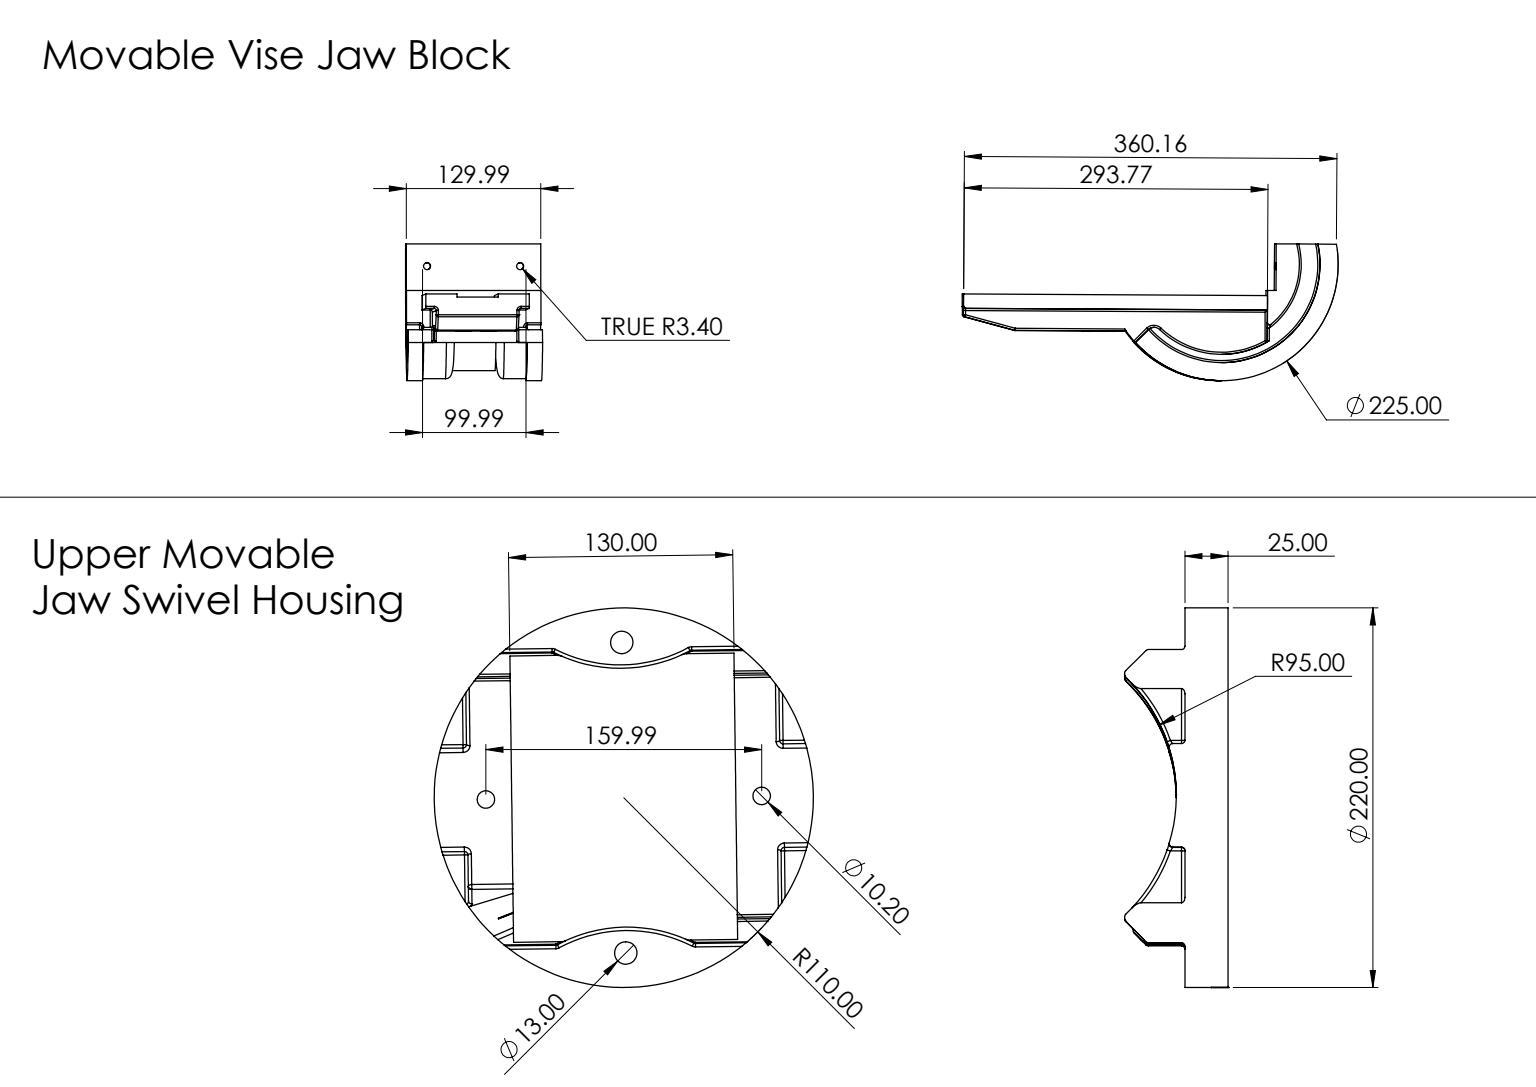
ISO-10303-21;
HEADER;
FILE_DESCRIPTION (('STEP AP214'),
    '1' );
FILE_NAME ('Movable Vise Jaw Block.step',
    '2026-10-09T10:51:02',
    ( '' ),
    ( '' ),
    'SwSTEP 2.0',
    'SolidWorks 2026',
    '' );
FILE_SCHEMA (( 'AUTOMOTIVE_DESIGN' ));
ENDSEC;

DATA;
#3=FACE_BOUND ( 'NONE', #13638, .T. ) ;
#7=LINE ( 'NONE', #21024, #14851 ) ;
#9=DIRECTION ( 'NONE',  ( 0.01292394549866739996, 0.005513023399721564584, 0.9999012842304692006 ) ) ;
#20=DIRECTION ( 'NONE',  ( 0.9999164797902017066, 6.965998958219365988E-18, -0.01292414190464157356 ) ) ;
#23=ORIENTED_EDGE ( 'NONE', *, *, #4860, .T. ) ;
#32=EDGE_CURVE ( 'NONE', #7434, #9119, #18827, .T. ) ;
#56=CARTESIAN_POINT ( 'NONE',  ( -66.42677970909001317, 189.3893605493459233, -109.9672025422466959 ) ) ;
#62=EDGE_CURVE ( 'NONE', #12374, #18464, #11714, .T. ) ;
#74=ORIENTED_EDGE ( 'NONE', *, *, #20006, .F. ) ;
#82=AXIS2_PLACEMENT_3D ( 'NONE', #13509, #3038, #10060 ) ;
#96=CARTESIAN_POINT ( 'NONE',  ( -45.67464185259402853, 168.2105890667581605, -51.90496219196452188 ) ) ;
#109=DIRECTION ( 'NONE',  ( -0.01292394549866736179, -0.005513023399728320464, -0.9999012842304692006 ) ) ;
#113=CONICAL_SURFACE ( 'NONE', #10017, 3.399999999999985700, 1.029744258676653201 ) ;
#115=ORIENTED_EDGE ( 'NONE', *, *, #3028, .T. ) ;
#117=CARTESIAN_POINT ( 'NONE',  ( -39.93340742419142941, 174.9483409995870886, 5.410635606648346752 ) ) ;
#119=CARTESIAN_POINT ( 'NONE',  ( -49.95600144165727841, 95.32463374251413768, -43.99660977802226114 ) ) ;
#124=CIRCLE ( 'NONE', #10026, 112.5000000000000142 ) ;
#136=AXIS2_PLACEMENT_3D ( 'NONE', #9103, #21501, #2221 ) ;
#140=DIRECTION ( 'NONE',  ( 0.9999164797902015955, 6.965998958219364448E-18, -0.01292414190464157182 ) ) ;
#141=CARTESIAN_POINT ( 'NONE',  ( 43.08423624159371457, 94.48610424851698042, 82.84014869562157912 ) ) ;
#148=CARTESIAN_POINT ( 'NONE',  ( -65.67129704762463405, 144.7109461922390778, -51.51693412452669918 ) ) ;
#149=AXIS2_PLACEMENT_3D ( 'NONE', #2906, #22065, #6366 ) ;
#163=VERTEX_POINT ( 'NONE', #8594 ) ;
#169=EDGE_CURVE ( 'NONE', #21645, #1999, #4525, .T. ) ;
#175=VECTOR ( 'NONE', #4968, 999.9999999999998863 ) ;
#178=CARTESIAN_POINT ( 'NONE',  ( -38.71484115365228007, 95.23700578170286235, 83.13812943312275650 ) ) ;
#185=CARTESIAN_POINT ( 'NONE',  ( -10.80196055862741211, 113.7230284608895943, 131.4548877534794542 ) ) ;
#187=ORIENTED_EDGE ( 'NONE', *, *, #11712, .T. ) ;
#193=CIRCLE ( 'NONE', #21802, 95.00000000000001421 ) ;
#208=ADVANCED_FACE ( 'NONE', ( #17222 ), #15410, .F. ) ;
#212=AXIS2_PLACEMENT_3D ( 'NONE', #480, #21365, #21476 ) ;
#229=ORIENTED_EDGE ( 'NONE', *, *, #7447, .T. ) ;
#238=DIRECTION ( 'NONE',  ( 0.01246513159389400598, 0.2641402835564878870, 0.9644037178988087433 ) ) ;
#241=ORIENTED_EDGE ( 'NONE', *, *, #10232, .T. ) ;
#242=CARTESIAN_POINT ( 'NONE',  ( -29.42617654240078551, 169.3906321239456361, -110.1596432836334856 ) ) ;
#245=ORIENTED_EDGE ( 'NONE', *, *, #7257, .T. ) ;
#257=ORIENTED_EDGE ( 'NONE', *, *, #16631, .F. ) ;
#262=DIRECTION ( 'NONE',  ( -0.01292394549866739996, -0.005513023399721131770, -0.9999012842304692006 ) ) ;
#263=CARTESIAN_POINT ( 'NONE',  ( -39.11958398656035030, 107.9174803907495885, 72.42004164600064087 ) ) ;
#264=DIRECTION ( 'NONE',  ( -7.125109674159588039E-05, 0.9999848031710253382, -0.005512562950848870491 ) ) ;
#269=EDGE_LOOP ( 'NONE', ( #10049, #17678 ) ) ;
#276=FACE_OUTER_BOUND ( 'NONE', #812, .T. ) ;
#280=CARTESIAN_POINT ( 'NONE',  ( -38.57134427488318806, 95.07266577213218284, 83.30245068639356987 ) ) ;
#286=ORIENTED_EDGE ( 'NONE', *, *, #7951, .T. ) ;
#292=EDGE_CURVE ( 'NONE', #16435, #21883, #7077, .T. ) ;
#296=B_SPLINE_CURVE_WITH_KNOTS ( 'NONE', 3,
 ( #20681, #1405, #18731, #13805, #4936, #18621, #1059, #11969, #4819, #17038, #18953, #20788, #17137, #20446, #8179, #13473 ),
 .UNSPECIFIED., .F., .F.,
 ( 4, 2, 2, 2, 2, 2, 2, 4 ),
 ( 0.000000000000000000, 0.0008474927940828290429, 0.001271239191124224699, 0.001694985588165620572, 0.002118731985207016229, 0.002542478382248412102, 0.002966224779289807541, 0.003389971176331203415 ),
 .UNSPECIFIED. ) ;
#302=DIRECTION ( 'NONE',  ( 0.01292394549866740169, 0.005513023399720822990, 0.9999012842304693116 ) ) ;
#309=VERTEX_POINT ( 'NONE', #21424 ) ;
#311=DIRECTION ( 'NONE',  ( 0.01292394549866739996, 0.005513023399721131770, 0.9999012842304692006 ) ) ;
#312=EDGE_LOOP ( 'NONE', ( #22638, #21700, #16864 ) ) ;
#329=CIRCLE ( 'NONE', #7287, 112.5000000000000284 ) ;
#332=VECTOR ( 'NONE', #8959, 1000.000000000000114 ) ;
#335=CARTESIAN_POINT ( 'NONE',  ( -66.44851505496320954, 169.3797848675314128, -111.6488252521261160 ) ) ;
#336=LINE ( 'NONE', #12856, #8327 ) ;
#338=CARTESIAN_POINT ( 'NONE',  ( -50.59154831888564274, 96.21415597129798414, -45.44386052779758245 ) ) ;
#340=CARTESIAN_POINT ( 'NONE',  ( -48.94038278341281512, 95.51270090492249665, 82.30370228625183415 ) ) ;
#344=ORIENTED_EDGE ( 'NONE', *, *, #10316, .T. ) ;
#346=CARTESIAN_POINT ( 'NONE',  ( 40.57355171551004958, 108.0982075334647163, 198.8652726751216449 ) ) ;
#374=CYLINDRICAL_SURFACE ( 'NONE', #1941, 2.000000000000001332 ) ;
#375=DIRECTION ( 'NONE',  ( 0.01292394549866743812, 0.005513023399720639109, 0.9999012842304693116 ) ) ;
#376=AXIS2_PLACEMENT_3D ( 'NONE', #2393, #7090, #10992 ) ;
#384=VECTOR ( 'NONE', #9453, 1000.000000000000000 ) ;
#395=CARTESIAN_POINT ( 'NONE',  ( -38.29718547875438617, 94.85299739018206822, 83.52102959496109236 ) ) ;
#411=ORIENTED_EDGE ( 'NONE', *, *, #12797, .F. ) ;
#413=ORIENTED_EDGE ( 'NONE', *, *, #15984, .T. ) ;
#415=DIRECTION ( 'NONE',  ( 0.01292394549866743812, 0.005513023399720639109, 0.9999012842304693116 ) ) ;
#424=AXIS2_PLACEMENT_3D ( 'NONE', #22195, #15240, #6485 ) ;
#427=ORIENTED_EDGE ( 'NONE', *, *, #15678, .F. ) ;
#436=AXIS2_PLACEMENT_3D ( 'NONE', #15343, #18765, #6586 ) ;
#444=VERTEX_POINT ( 'NONE', #19641 ) ;
#446=AXIS2_PLACEMENT_3D ( 'NONE', #5917, #9248, #537 ) ;
#451=EDGE_CURVE ( 'NONE', #8312, #552, #9105, .T. ) ;
#470=CARTESIAN_POINT ( 'NONE',  ( 40.93042701181084908, 108.3156947416822362, 71.72688916598494302 ) ) ;
#473=ORIENTED_EDGE ( 'NONE', *, *, #11263, .F. ) ;
#480=CARTESIAN_POINT ( 'NONE',  ( -49.99582398951010731, 170.0000000000000284, 0.6462070952320568828 ) ) ;
#481=AXIS2_PLACEMENT_3D ( 'NONE', #12195, #19178, #15648 ) ;
#494=CARTESIAN_POINT ( 'NONE',  ( 40.97039650227475249, 106.5772003501581082, 92.39653500429078292 ) ) ;
#498=DIRECTION ( 'NONE',  ( -0.01292394549866743465, -0.005513023399716638837, -0.9999012842304692006 ) ) ;
#499=ORIENTED_EDGE ( 'NONE', *, *, #15162, .T. ) ;
#508=DIRECTION ( 'NONE',  ( -0.9999164797902015955, -6.965998958219364448E-18, 0.01292414190464157182 ) ) ;
#511=EDGE_CURVE ( 'NONE', #21004, #6936, #16422, .T. ) ;
#520=CARTESIAN_POINT ( 'NONE',  ( -48.91844876508264406, 94.45452722259994971, 84.00069590936301722 ) ) ;
#532=EDGE_CURVE ( 'NONE', #9660, #4358, #8369, .T. ) ;
#533=AXIS2_PLACEMENT_3D ( 'NONE', #8570, #17553, #22151 ) ;
#534=CIRCLE ( 'NONE', #5661, 7.921742784567035400 ) ;
#537=DIRECTION ( 'NONE',  ( -7.125109674243555432E-05, 0.9999848031710253382, -0.005512562950850175003 ) ) ;
#546=DIRECTION ( 'NONE',  ( -7.125109674159588039E-05, 0.9999848031710253382, -0.005512562950848870491 ) ) ;
#547=ADVANCED_FACE ( 'NONE', ( #15195 ), #4588, .F. ) ;
#548=CARTESIAN_POINT ( 'NONE',  ( 51.68650743418692173, 107.0878900929417057, 69.97116258175249470 ) ) ;
#552=VERTEX_POINT ( 'NONE', #13353 ) ;
#563=AXIS2_PLACEMENT_3D ( 'NONE', #12905, #21489, #12783 ) ;
#570=DIRECTION ( 'NONE',  ( -0.01292394549866736179, -0.005513023399721110954, -0.9999012842304692006 ) ) ;
#574=ORIENTED_EDGE ( 'NONE', *, *, #16977, .F. ) ;
#582=CARTESIAN_POINT ( 'NONE',  ( -49.99268894125347629, 126.0006686604749291, 0.8887598650694636948 ) ) ;
#587=CARTESIAN_POINT ( 'NONE',  ( 42.39538333684826910, 106.8539349815730333, 70.43383574752205334 ) ) ;
#590=VECTOR ( 'NONE', #9776, 1000.000000000000114 ) ;
#594=PLANE ( 'NONE',  #11466 ) ;
#604=CARTESIAN_POINT ( 'NONE',  ( 49.71850332751439083, 189.5983039071083738, -73.56585792680235159 ) ) ;
#606=FACE_OUTER_BOUND ( 'NONE', #18445, .T. ) ;
#608=CARTESIAN_POINT ( 'NONE',  ( -40.94748323230124498, 106.8060942374655298, 71.46846058825224191 ) ) ;
#610=CARTESIAN_POINT ( 'NONE',  ( -50.62910760614470718, 109.0971227715196363, -45.77181594070039239 ) ) ;
#611=ORIENTED_EDGE ( 'NONE', *, *, #32, .F. ) ;
#622=CARTESIAN_POINT ( 'NONE',  ( -38.35540033123504600, 106.2286129618570243, 92.30320912117649357 ) ) ;
#634=CARTESIAN_POINT ( 'NONE',  ( 49.06020240426833112, 189.6011917897851333, -73.03348424162913943 ) ) ;
#639=AXIS2_PLACEMENT_3D ( 'NONE', #5949, #21340, #11248 ) ;
#645=CARTESIAN_POINT ( 'NONE',  ( 49.99582398951007889, 170.0000000000000284, -0.6462070952321007367 ) ) ;
#649=EDGE_CURVE ( 'NONE', #10347, #7226, #17734, .T. ) ;
#665=VERTEX_POINT ( 'NONE', #6769 ) ;
#679=CIRCLE ( 'NONE', #12037, 112.5000000000007105 ) ;
#684=ORIENTED_EDGE ( 'NONE', *, *, #11712, .F. ) ;
#690=ORIENTED_EDGE ( 'NONE', *, *, #4006, .F. ) ;
#701=DIRECTION ( 'NONE',  ( -0.01292394549866744159, -0.005513023399721241925, -0.9999012842304693116 ) ) ;
#703=ORIENTED_EDGE ( 'NONE', *, *, #10621, .T. ) ;
#710=EDGE_CURVE ( 'NONE', #8991, #1318, #19167, .T. ) ;
#713=CARTESIAN_POINT ( 'NONE',  ( 18.67136755788715519, 169.4339520569534159, -102.9230326054181290 ) ) ;
#714=CARTESIAN_POINT ( 'NONE',  ( 51.06003536384874053, 189.6011917897851333, -73.05933252543843537 ) ) ;
#719=VERTEX_POINT ( 'NONE', #21007 ) ;
#721=DIRECTION ( 'NONE',  ( -0.9999164797902015955, -6.965998958219364448E-18, 0.01292414190464157182 ) ) ;
#726=VERTEX_POINT ( 'NONE', #19511 ) ;
#741=CARTESIAN_POINT ( 'NONE',  ( -37.45866066553108453, 94.51302055746239716, 83.85396645971145801 ) ) ;
#759=DIRECTION ( 'NONE',  ( -0.9999164797902015955, -6.965998958219364448E-18, 0.01292414190464157182 ) ) ;
#764=DIRECTION ( 'NONE',  ( 0.01292394549866739996, 0.005513023399721131770, 0.9999012842304692006 ) ) ;
#774=CARTESIAN_POINT ( 'NONE',  ( -41.99649215118849810, 170.0000000000000284, 0.5428139599949243221 ) ) ;
#783=ORIENTED_EDGE ( 'NONE', *, *, #14046, .T. ) ;
#785=AXIS2_PLACEMENT_3D ( 'NONE', #7966, #15001, #20026 ) ;
#793=CARTESIAN_POINT ( 'NONE',  ( 20.96603472858062034, 99.74539563421257071, 74.61103786048234099 ) ) ;
#801=ORIENTED_EDGE ( 'NONE', *, *, #7186, .T. ) ;
#804=AXIS2_PLACEMENT_3D ( 'NONE', #2350, #11419, #18214 ) ;
#811=ADVANCED_FACE ( 'NONE', ( #12645 ), #19833, .T. ) ;
#812=EDGE_LOOP ( 'NONE', ( #5631, #6590, #17195, #4960 ) ) ;
#823=CARTESIAN_POINT ( 'NONE',  ( -41.99335710293186708, 126.0006686604749291, 0.7853667298323311341 ) ) ;
#824=CARTESIAN_POINT ( 'NONE',  ( -52.30302070948153670, 110.0041276461028019, -43.49757385923464170 ) ) ;
#835=FACE_OUTER_BOUND ( 'NONE', #10421, .T. ) ;
#848=VERTEX_POINT ( 'NONE', #12748 ) ;
#850=VERTEX_POINT ( 'NONE', #21454 ) ;
#853=EDGE_CURVE ( 'NONE', #7530, #5831, #12014, .T. ) ;
#863=CARTESIAN_POINT ( 'NONE',  ( -38.89440990870000547, 93.50952370771440769, 84.88723154575897922 ) ) ;
#864=EDGE_CURVE ( 'NONE', #9499, #6519, #336, .T. ) ;
#870=PLANE ( 'NONE',  #804 ) ;
#879=CARTESIAN_POINT ( 'NONE',  ( 42.27543525282722214, 106.8832415124691977, 70.46146445762853716 ) ) ;
#881=EDGE_CURVE ( 'NONE', #10347, #20680, #7329, .T. ) ;
#883=VERTEX_POINT ( 'NONE', #12988 ) ;
#884=CARTESIAN_POINT ( 'NONE',  ( -50.60913278034716001, 111.9218655255082382, -46.80433714073992491 ) ) ;
#887=LINE ( 'NONE', #12824, #12247 ) ;
#889=ORIENTED_EDGE ( 'NONE', *, *, #21935, .T. ) ;
#892=DIRECTION ( 'NONE',  ( -0.9999164797902017066, -6.965998958219367529E-18, 0.01292414190464157182 ) ) ;
#910=LINE ( 'NONE', #4658, #15177 ) ;
#911=DIRECTION ( 'NONE',  ( -0.01292394549866740863, -0.005513023399721009472, -0.9999012842304692006 ) ) ;
#920=CARTESIAN_POINT ( 'NONE',  ( 64.99457118636310327, 170.0000000000000284, -0.8400692238017243296 ) ) ;
#934=DIRECTION ( 'NONE',  ( -0.01292394549866740169, -0.005513023399721021615, -0.9999012842304692006 ) ) ;
#935=CARTESIAN_POINT ( 'NONE',  ( -51.81471661454150279, 109.8909348587996817, -43.50326120169058441 ) ) ;
#944=ADVANCED_FACE ( 'NONE', ( #2510 ), #2163, .T. ) ;
#946=DIRECTION ( 'NONE',  ( -0.9999164797902015955, -6.965998958219364448E-18, 0.01292414190464157182 ) ) ;
#951=CARTESIAN_POINT ( 'NONE',  ( -38.57295527635426424, 106.5467666792623760, 92.13836866384394853 ) ) ;
#953=ORIENTED_EDGE ( 'NONE', *, *, #4737, .T. ) ;
#956=VERTEX_POINT ( 'NONE', #16545 ) ;
#961=DIRECTION ( 'NONE',  ( -0.01292394549866695240, -0.005513023399718316314, -0.9999012842304693116 ) ) ;
#969=CARTESIAN_POINT ( 'NONE',  ( -37.89664629966064524, 96.09134658471360524, 84.97026380959019320 ) ) ;
#978=ADVANCED_FACE ( 'NONE', ( #5088 ), #11660, .F. ) ;
#985=CARTESIAN_POINT ( 'NONE',  ( 41.70036908154883548, 107.1149823552813700, 70.67426363338570638 ) ) ;
#990=DIRECTION ( 'NONE',  ( -0.01292394549866737741, -0.005513023399721125699, -0.9999012842304693116 ) ) ;
#997=CARTESIAN_POINT ( 'NONE',  ( -40.44015661483791035, 106.8832415124692545, 71.53058179755718982 ) ) ;
#999=ADVANCED_FACE ( 'NONE', ( #4981 ), #4446, .F. ) ;
#1004=CARTESIAN_POINT ( 'NONE',  ( 49.90104868606460542, 189.4888640791102716, -93.42071897647797130 ) ) ;
#1005=ORIENTED_EDGE ( 'NONE', *, *, #18216, .T. ) ;
#1011=CARTESIAN_POINT ( 'NONE',  ( -46.79684245571608869, 129.3639651298425406, 248.1453739866443868 ) ) ;
#1029=PRODUCT_DEFINITION ( 'UNKNOWN', '', #9172, #1464 ) ;
#1032=AXIS2_PLACEMENT_3D ( 'NONE', #9960, #10081, #17093 ) ;
#1034=FACE_OUTER_BOUND ( 'NONE', #22468, .T. ) ;
#1035=CARTESIAN_POINT ( 'NONE',  ( -48.90389017660277915, 110.4330569016835852, -43.54387330449551996 ) ) ;
#1053=EDGE_CURVE ( 'NONE', #19370, #9718, #14609, .T. ) ;
#1059=CARTESIAN_POINT ( 'NONE',  ( 48.97873930546568033, 95.44197026330519407, -45.47108626627597516 ) ) ;
#1062=ORIENTED_EDGE ( 'NONE', *, *, #4292, .F. ) ;
#1069=EDGE_CURVE ( 'NONE', #7401, #8679, #22404, .T. ) ;
#1080=ORIENTED_EDGE ( 'NONE', *, *, #1116, .T. ) ;
#1084=DIRECTION ( 'NONE',  ( 0.000000000000000000, -0.005512562964840580192, -0.9999848057093461140 ) ) ;
#1092=ORIENTED_EDGE ( 'NONE', *, *, #864, .T. ) ;
#1106=CARTESIAN_POINT ( 'NONE',  ( -20.57109388430227881, 136.7551719540686008, -44.05520973278501629 ) ) ;
#1111=CARTESIAN_POINT ( 'NONE',  ( 42.07978785083213324, 94.68322439548107639, 83.03125727779237764 ) ) ;
#1115=AXIS2_PLACEMENT_3D ( 'NONE', #19056, #18843, #4694 ) ;
#1116=EDGE_CURVE ( 'NONE', #4358, #13904, #17148, .T. ) ;
#1120=EDGE_LOOP ( 'NONE', ( #22490, #2558, #19799, #17499, #8659 ) ) ;
#1121=CARTESIAN_POINT ( 'NONE',  ( 48.91192295135010681, 189.4953846123264611, -92.22510262217610943 ) ) ;
#1124=AXIS2_PLACEMENT_3D ( 'NONE', #11235, #22101, #13312 ) ;
#1130=DIRECTION ( 'NONE',  ( 0.9999164797902015955, 6.965998958219364448E-18, -0.01292414190464157182 ) ) ;
#1133=CARTESIAN_POINT ( 'NONE',  ( 64.99457118636310327, 170.0000000000000284, -0.8400692238017243296 ) ) ;
#1139=EDGE_CURVE ( 'NONE', #5652, #18473, #9821, .T. ) ;
#1143=CARTESIAN_POINT ( 'NONE',  ( 64.39761729661502443, 113.4706157781613598, -47.02526561348111755 ) ) ;
#1145=ORIENTED_EDGE ( 'NONE', *, *, #5482, .T. ) ;
#1152=CIRCLE ( 'NONE', #424, 3.399999999999985700 ) ;
#1158=ADVANCED_FACE ( 'NONE', ( #10937 ), #19649, .T. ) ;
#1161=CIRCLE ( 'NONE', #13994, 112.5000000000007105 ) ;
#1162=CARTESIAN_POINT ( 'NONE',  ( -52.89202980190114545, 109.4892200475068904, -43.48712180841023667 ) ) ;
#1163=DIRECTION ( 'NONE',  ( -0.9999164797902015955, -6.965998958219364448E-18, 0.01292414190464157182 ) ) ;
#1203=CARTESIAN_POINT ( 'NONE',  ( -52.29989087310946871, 189.4888611505737117, -92.10028044281781945 ) ) ;
#1204=ORIENTED_EDGE ( 'NONE', *, *, #4008, .F. ) ;
#1207=CARTESIAN_POINT ( 'NONE',  ( 18.69536052806380866, 189.4444907833431273, -101.0667417618365107 ) ) ;
#1215=( BOUNDED_SURFACE ( )  B_SPLINE_SURFACE ( 3, 2, ( 
 ( #2977, #9995, #11265 ),
 ( #22144, #4348, #14957 ),
 ( #13453, #11375, #18275 ),
 ( #2534, #13227, #9535 ),
 ( #18385, #1162, #21908 ),
 ( #17020, #1284, #18707 ),
 ( #14737, #8157, #20323 ),
 ( #21690, #6327, #11610 ),
 ( #5975, #13014, #2653 ),
 ( #19974, #2764, #4243 ),
 ( #16571, #824, #7818 ),
 ( #14853, #6087, #13346 ),
 ( #9663, #935, #4468 ),
 ( #16691, #6200, #11497 ),
 ( #18503, #9772, #1035 ),
 ( #4581, #2864, #10554 ),
 ( #8267, #22248, #13785 ),
 ( #3540, #17576, #15630 ),
 ( #5138, #18831, #12176 ),
 ( #4797, #19043, #15519 ) ),
 .UNSPECIFIED., .F., .F., .T. ) 
 B_SPLINE_SURFACE_WITH_KNOTS ( ( 4, 2, 2, 2, 2, 2, 2, 2, 2, 4 ),
 ( 3, 3 ),
 ( 0.002250506978132263327, 0.003145136895573769423, 0.003592451854294522254, 0.004039766813015275085, 0.004934396730456780747, 0.005829026647898287276, 0.006723656565339793806, 0.007618286482781299468, 0.008512916400222805130, 0.009407546317664310792 ),
 ( 0.000000000000000000, 1.000000000000000000 ),
 .UNSPECIFIED. ) 
 GEOMETRIC_REPRESENTATION_ITEM ( )  RATIONAL_B_SPLINE_SURFACE ( (
 ( 1.000000000000000000, 0.4260362065776441831, 1.000000000000000000),
 ( 1.000000000000000000, 0.4260393075400374374, 1.000000000000000000),
 ( 1.000000000000000000, 0.4294086899200588170, 1.000000000000000000),
 ( 1.000000000000000000, 0.4387845791473878876, 1.000000000000000000),
 ( 1.000000000000000000, 0.4426643443719024407, 1.000000000000000000),
 ( 1.000000000000000000, 0.4514921189388687028, 1.000000000000000000),
 ( 1.000000000000000000, 0.4564487767892564385, 1.000000000000000000),
 ( 1.000000000000000000, 0.4726420716812023137, 1.000000000000000000),
 ( 1.000000000000000000, 0.4853216829651075814, 1.000000000000000000),
 ( 1.000000000000000000, 0.5119006064974717107, 1.000000000000000000),
 ( 1.000000000000000000, 0.5258950471250586345, 1.000000000000000000),
 ( 1.000000000000000000, 0.5546623498312363010, 1.000000000000000000),
 ( 1.000000000000000000, 0.5692926216424040176, 1.000000000000000000),
 ( 1.000000000000000000, 0.5980609968324860359, 1.000000000000000000),
 ( 1.000000000000000000, 0.6123199638066775252, 1.000000000000000000),
 ( 1.000000000000000000, 0.6405585493648041640, 1.000000000000000000),
 ( 1.000000000000000000, 0.6545126017561364584, 1.000000000000000000),
 ( 1.000000000000000000, 0.6813871835234406316, 1.000000000000000000),
 ( 1.000000000000000000, 0.6944185932103925651, 1.000000000000000000),
 ( 1.000000000000000000, 0.7071067811865477948, 1.000000000000000000) ) ) 
 REPRESENTATION_ITEM ( '' )  SURFACE ( )  );
#1221=ORIENTED_EDGE ( 'NONE', *, *, #3881, .T. ) ;
#1228=CARTESIAN_POINT ( 'NONE',  ( -50.55759505772823559, 106.8515392057802273, 71.54635382116403264 ) ) ;
#1231=CARTESIAN_POINT ( 'NONE',  ( -48.91807906390275207, 94.48610424851698042, 84.02929899226764121 ) ) ;
#1236=TOROIDAL_SURFACE ( 'NONE', #4869, 9.921742784567035400, 2.000000000000000000 ) ;
#1238=CIRCLE ( 'NONE', #481, 77.00000000000002842 ) ;
#1246=CARTESIAN_POINT ( 'NONE',  ( -37.61323352684398458, 61.62499466978435692, 30.16896140480725208 ) ) ;
#1250=CARTESIAN_POINT ( 'NONE',  ( 19.42535155401557390, 139.7551263635816952, -44.58871309782322356 ) ) ;
#1266=DIRECTION ( 'NONE',  ( 0.9999164797902015955, 6.965998958219364448E-18, -0.01292414190464157182 ) ) ;
#1267=VECTOR ( 'NONE', #14434, 1000.000000000000114 ) ;
#1268=ORIENTED_EDGE ( 'NONE', *, *, #21818, .F. ) ;
#1277=CARTESIAN_POINT ( 'NONE',  ( -10.85567112094788200, 105.6999953372425409, 127.2994028633183063 ) ) ;
#1284=CARTESIAN_POINT ( 'NONE',  ( -52.89610439416505727, 109.5992314273289026, -43.48767569858423343 ) ) ;
#1287=LINE ( 'NONE', #22357, #13681 ) ;
#1289=CARTESIAN_POINT ( 'NONE',  ( 41.20572975695933593, 107.5148010522800064, 93.02654324256212703 ) ) ;
#1290=CARTESIAN_POINT ( 'NONE',  ( 65.76886434875187604, 106.9149828242082947, 59.06553216729307110 ) ) ;
#1303=CIRCLE ( 'NONE', #11193, 2.000000000000001332 ) ;
#1304=CARTESIAN_POINT ( 'NONE',  ( -66.44851505496320954, 169.3797848675314128, -111.6488252521261160 ) ) ;
#1307=CARTESIAN_POINT ( 'NONE',  ( 41.19638261157623305, 121.2962013336460814, 247.0525242307099347 ) ) ;
#1313=DIRECTION ( 'NONE',  ( -0.01292394549866739822, -0.005513023399721269681, -0.9999012842304692006 ) ) ;
#1317=CARTESIAN_POINT ( 'NONE',  ( -51.24077369867691800, 189.4960777121730473, -90.80487779002250193 ) ) ;
#1318=VERTEX_POINT ( 'NONE', #2778 ) ;
#1327=AXIS2_PLACEMENT_3D ( 'NONE', #18507, #7930, #13351 ) ;
#1328=CARTESIAN_POINT ( 'NONE',  ( 44.03004128744986190, 171.4878726268958360, -75.33468125154308836 ) ) ;
#1334=ORIENTED_EDGE ( 'NONE', *, *, #18596, .F. ) ;
#1337=AXIS2_PLACEMENT_3D ( 'NONE', #19395, #892, #13182 ) ;
#1341=ORIENTED_EDGE ( 'NONE', *, *, #10232, .F. ) ;
#1353=ORIENTED_EDGE ( 'NONE', *, *, #7238, .T. ) ;
#1355=EDGE_LOOP ( 'NONE', ( #16218, #8476, #413, #7161 ) ) ;
#1365=VERTEX_POINT ( 'NONE', #13243 ) ;
#1372=EDGE_CURVE ( 'NONE', #16531, #4876, #8378, .T. ) ;
#1381=AXIS2_PLACEMENT_3D ( 'NONE', #18157, #9162, #7454 ) ;
#1393=CARTESIAN_POINT ( 'NONE',  ( 51.76881283800809541, 109.6007514900105093, -44.84050130987714056 ) ) ;
#1395=DIRECTION ( 'NONE',  ( 1.000000000000000000, 0.000000000000000000, 0.000000000000000000 ) ) ;
#1404=ORIENTED_EDGE ( 'NONE', *, *, #20725, .T. ) ;
#1405=CARTESIAN_POINT ( 'NONE',  ( 49.40325090546203057, 96.06183802811887062, -46.49246881160556910 ) ) ;
#1406=DIRECTION ( 'NONE',  ( -0.01292394549866736873, -0.005513023399721228915, -0.9999012842304690896 ) ) ;
#1417=CARTESIAN_POINT ( 'NONE',  ( 42.77078531357724245, 106.9149828242082947, 59.36278743109983225 ) ) ;
#1420=CARTESIAN_POINT ( 'NONE',  ( 44.31808358225305966, 164.8106407359766763, -53.04939224934937414 ) ) ;
#1421=CARTESIAN_POINT ( 'NONE',  ( -51.17105351027176141, 189.4989811950858609, -90.27908403945292548 ) ) ;
#1435=CARTESIAN_POINT ( 'NONE',  ( 41.42451162475439475, 125.7553391191873544, -44.79586833841344173 ) ) ;
#1437=ORIENTED_EDGE ( 'NONE', *, *, #8759, .T. ) ;
#1441=EDGE_CURVE ( 'NONE', #21136, #10347, #7244, .T. ) ;
#1453=DIRECTION ( 'NONE',  ( -0.009088227368120101179, -0.7109943316365099353, -0.7031390079522383818 ) ) ;
#1454=ORIENTED_EDGE ( 'NONE', *, *, #16589, .T. ) ;
#1457=CARTESIAN_POINT ( 'NONE',  ( -37.38389485984217941, 95.54566594239412325, 84.82795484212111603 ) ) ;
#1462=ORIENTED_EDGE ( 'NONE', *, *, #2047, .F. ) ;
#1463=LINE ( 'NONE', #4552, #13309 ) ;
#1464=PRODUCT_DEFINITION_CONTEXT ( 'detailed design', #20253, 'design' ) ;
#1494=CARTESIAN_POINT ( 'NONE',  ( 64.99457118636310327, 170.0000000000000284, -0.8400692238017243296 ) ) ;
#1502=CARTESIAN_POINT ( 'NONE',  ( 49.81003579750536403, 110.5281110817785049, -47.59029815665551411 ) ) ;
#1505=AXIS2_PLACEMENT_3D ( 'NONE', #20426, #11715, #2979 ) ;
#1507=CARTESIAN_POINT ( 'NONE',  ( -48.59258154118273865, 108.3707227317548529, -45.53672366955343165 ) ) ;
#1509=EDGE_CURVE ( 'NONE', #848, #22315, #10189, .T. ) ;
#1527=CARTESIAN_POINT ( 'NONE',  ( -34.80083724429680814, 171.3633268630252644, 247.7587566398530612 ) ) ;
#1547=CARTESIAN_POINT ( 'NONE',  ( 47.42517700970201133, 109.3838229944194609, -44.78316280508298775 ) ) ;
#1557=PLANE ( 'NONE',  #13925 ) ;
#1571=VERTEX_POINT ( 'NONE', #2067 ) ;
#1576=AXIS2_PLACEMENT_3D ( 'NONE', #20398, #18806, #9968 ) ;
#1593=CIRCLE ( 'NONE', #11489, 2.000000000000005329 ) ;
#1599=LINE ( 'NONE', #5474, #11835 ) ;
#1601=CARTESIAN_POINT ( 'NONE',  ( 18.69536052806381576, 189.4444907833431273, -101.0667417618364965 ) ) ;
#1607=CARTESIAN_POINT ( 'NONE',  ( 64.42259306105445660, 139.7551263635816952, -45.17031240767400391 ) ) ;
#1610=ORIENTED_EDGE ( 'NONE', *, *, #13094, .F. ) ;
#1612=AXIS2_PLACEMENT_3D ( 'NONE', #16636, #16404, #21423 ) ;
#1621=DIRECTION ( 'NONE',  ( -7.125109674243555432E-05, 0.9999848031710253382, -0.005512562950850175003 ) ) ;
#1625=EDGE_LOOP ( 'NONE', ( #5052, #16017, #17901, #17803 ) ) ;
#1635=EDGE_LOOP ( 'NONE', ( #7699, #12746 ) ) ;
#1637=FACE_OUTER_BOUND ( 'NONE', #10344, .T. ) ;
#1639=CIRCLE ( 'NONE', #20337, 110.5324305509042233 ) ;
#1642=DIRECTION ( 'NONE',  ( -0.9999164797902015955, -6.965998958219364448E-18, 0.01292414190464157182 ) ) ;
#1650=CARTESIAN_POINT ( 'NONE',  ( -40.73497377069196546, 95.07629454920768808, 83.32674675967490430 ) ) ;
#1652=DIRECTION ( 'NONE',  ( 0.9999164797902015955, 6.965998958219364448E-18, -0.01292414190464157182 ) ) ;
#1664=VERTEX_POINT ( 'NONE', #17478 ) ;
#1681=ORIENTED_EDGE ( 'NONE', *, *, #19106, .T. ) ;
#1688=ORIENTED_EDGE ( 'NONE', *, *, #1509, .F. ) ;
#1697=CARTESIAN_POINT ( 'NONE',  ( 64.31463902574824942, 189.7102623349352086, -53.44513790491837568 ) ) ;
#1703=VERTEX_POINT ( 'NONE', #20071 ) ;
#1710=DIRECTION ( 'NONE',  ( -0.008899921406766564749, 0.7251151399516315710, -0.6885701309321218266 ) ) ;
#1711=CARTESIAN_POINT ( 'NONE',  ( 41.19649195735513558, 119.7615706795621691, 247.0609841073601842 ) ) ;
#1712=DIRECTION ( 'NONE',  ( 0.01292394549866739996, 0.005513023399721131770, 0.9999012842304692006 ) ) ;
#1713=CARTESIAN_POINT ( 'NONE',  ( 18.38499007693353349, 64.93155780410931754, -125.0795181004832415 ) ) ;
#1715=DIRECTION ( 'NONE',  ( 0.01292394549866740169, 0.005513023399720822990, 0.9999012842304693116 ) ) ;
#1737=LINE ( 'NONE', #17598, #21237 ) ;
#1745=VERTEX_POINT ( 'NONE', #14718 ) ;
#1750=ORIENTED_EDGE ( 'NONE', *, *, #1372, .T. ) ;
#1762=DIRECTION ( 'NONE',  ( 0.9999164797902015955, 6.965998958219364448E-18, -0.01292414190464157182 ) ) ;
#1763=ORIENTED_EDGE ( 'NONE', *, *, #15678, .T. ) ;
#1773=EDGE_CURVE ( 'NONE', #22552, #13067, #11786, .T. ) ;
#1785=DIRECTION ( 'NONE',  ( 0.9999164797902015955, 6.965998958219364448E-18, -0.01292414190464157182 ) ) ;
#1803=CARTESIAN_POINT ( 'NONE',  ( 50.89197640125190958, 108.0238286078847523, 68.68741454989820738 ) ) ;
#1816=DIRECTION ( 'NONE',  ( 0.01292394549866740169, 0.005513023399720822990, 0.9999012842304693116 ) ) ;
#1817=ADVANCED_FACE ( 'NONE', ( #5221 ), #10757, .F. ) ;
#1825=CARTESIAN_POINT ( 'NONE',  ( 49.65978088490153652, 110.1615718061116951, -47.45444771764796599 ) ) ;
#1826=ORIENTED_EDGE ( 'NONE', *, *, #4420, .F. ) ;
#1830=CARTESIAN_POINT ( 'NONE',  ( 49.39923347825703104, 108.3707227317548529, -46.80328957620832142 ) ) ;
#1832=LINE ( 'NONE', #20893, #14866 ) ;
#1835=VECTOR ( 'NONE', #19052, 999.9999999999998863 ) ;
#1849=VERTEX_POINT ( 'NONE', #22654 ) ;
#1861=AXIS2_PLACEMENT_3D ( 'NONE', #18672, #7651, #20052 ) ;
#1867=CARTESIAN_POINT ( 'NONE',  ( 39.45263645499988314, 96.15465585523027414, -42.60697859377187058 ) ) ;
#1875=VECTOR ( 'NONE', #19004, 1000.000000000000114 ) ;
#1889=AXIS2_PLACEMENT_3D ( 'NONE', #11521, #2787, #22378 ) ;
#1890=CARTESIAN_POINT ( 'NONE',  ( -38.70754582269196220, 96.72929363966481731, 84.40869485543453266 ) ) ;
#1899=EDGE_LOOP ( 'NONE', ( #5563, #2921, #4892, #3591 ) ) ;
#1913=CIRCLE ( 'NONE', #12565, 75.00000000000002842 ) ;
#1940=CIRCLE ( 'NONE', #12591, 77.00000000000002842 ) ;
#1941=AXIS2_PLACEMENT_3D ( 'NONE', #12342, #16027, #14182 ) ;
#1953=CARTESIAN_POINT ( 'NONE',  ( -48.85087316658617596, 95.00692584804919250, -43.47488344668517612 ) ) ;
#1954=ORIENTED_EDGE ( 'NONE', *, *, #17504, .T. ) ;
#1956=DIRECTION ( 'NONE',  ( -0.01292394549866743465, -0.005513023399721021615, -0.9999012842304692006 ) ) ;
#1961=AXIS2_PLACEMENT_3D ( 'NONE', #5271, #6777, #12316 ) ;
#1966=EDGE_CURVE ( 'NONE', #9119, #13016, #18107, .T. ) ;
#1968=AXIS2_PLACEMENT_3D ( 'NONE', #15363, #22311, #17298 ) ;
#1973=TOROIDAL_SURFACE ( 'NONE', #20288, 77.00000000000002842, 2.000000000000000000 ) ;
#1984=EDGE_CURVE ( 'NONE', #14056, #15010, #6897, .T. ) ;
#1990=CARTESIAN_POINT ( 'NONE',  ( 40.57369421770351892, 106.0982379271226677, 198.8762978010233553 ) ) ;
#1993=SURFACE_STYLE_USAGE ( .BOTH. , #12447 ) ;
#1997=VECTOR ( 'NONE', #15627, 1000.000000000000000 ) ;
#1999=VERTEX_POINT ( 'NONE', #17170 ) ;
#2006=CARTESIAN_POINT ( 'NONE',  ( 41.42670316190684332, 94.99786382055523859, -44.62631324292065926 ) ) ;
#2010=CARTESIAN_POINT ( 'NONE',  ( -40.52114077660952773, 94.71095003552228775, 83.69340898796828299 ) ) ;
#2025=DIRECTION ( 'NONE',  ( 0.01292394549866743812, 0.005513023399720639109, 0.9999012842304693116 ) ) ;
#2032=ORIENTED_EDGE ( 'NONE', *, *, #8503, .F. ) ;
#2040=ORIENTED_EDGE ( 'NONE', *, *, #14453, .T. ) ;
#2043=DIRECTION ( 'NONE',  ( -7.125109674243555432E-05, 0.9999848031710253382, -0.005512562950850175003 ) ) ;
#2047=EDGE_CURVE ( 'NONE', #22611, #2091, #8370, .T. ) ;
#2050=EDGE_CURVE ( 'NONE', #7916, #1999, #12117, .T. ) ;
#2057=ORIENTED_EDGE ( 'NONE', *, *, #3919, .F. ) ;
#2060=VERTEX_POINT ( 'NONE', #14306 ) ;
#2063=ORIENTED_EDGE ( 'NONE', *, *, #17873, .T. ) ;
#2067=CARTESIAN_POINT ( 'NONE',  ( -50.59154831888564274, 96.21415597129798414, -45.44386052779758245 ) ) ;
#2070=VERTEX_POINT ( 'NONE', #16151 ) ;
#2091=VERTEX_POINT ( 'NONE', #6924 ) ;
#2099=CARTESIAN_POINT ( 'NONE',  ( -10.95260071218788767, 105.6586476617446380, 119.8001432315898001 ) ) ;
#2100=EDGE_LOOP ( 'NONE', ( #20940, #11395, #17245, #7655, #16464, #6898, #6647, #17037, #21021, #783, #13454, #13565, #12886, #17622 ) ) ;
#2102=ORIENTED_EDGE ( 'NONE', *, *, #6323, .T. ) ;
#2112=CARTESIAN_POINT ( 'NONE',  ( -39.92320284967681232, 94.09382044627800212, 84.30970454134384795 ) ) ;
#2113=ADVANCED_FACE ( 'NONE', ( #17521 ), #17632, .T. ) ;
#2120=LINE ( 'NONE', #3729, #11025 ) ;
#2123=DIRECTION ( 'NONE',  ( -0.01292394549866695240, -0.005513023399725255208, -0.9999012842304693116 ) ) ;
#2151=ADVANCED_FACE ( 'NONE', ( #276 ), #5544, .T. ) ;
#2158=CARTESIAN_POINT ( 'NONE',  ( 41.19638261157624015, 121.2962013336460814, 247.0525242307099347 ) ) ;
#2161=EDGE_LOOP ( 'NONE', ( #15991, #9452, #19555, #18830 ) ) ;
#2163=CYLINDRICAL_SURFACE ( 'NONE', #1381, 1.999999999999998446 ) ;
#2164=CARTESIAN_POINT ( 'NONE',  ( -50.21426504490502651, 95.50261743988794194, -44.28974071693060210 ) ) ;
#2165=ORIENTED_EDGE ( 'NONE', *, *, #12912, .F. ) ;
#2166=DIRECTION ( 'NONE',  ( 0.9999164797902015955, 6.965998958219364448E-18, -0.01292414190464157182 ) ) ;
#2167=DIRECTION ( 'NONE',  ( 0.9999164797902015955, 6.965998958219364448E-18, -0.01292414190464157182 ) ) ;
#2170=VERTEX_POINT ( 'NONE', #14650 ) ;
#2171=CARTESIAN_POINT ( 'NONE',  ( -39.99665919160808869, 170.0000000000000284, 0.5169656761856410432 ) ) ;
#2202=CIRCLE ( 'NONE', #12498, 110.5324305509042233 ) ;
#2203=CARTESIAN_POINT ( 'NONE',  ( -51.08857079363052378, 110.6671980935713293, -46.33702760430572454 ) ) ;
#2221=DIRECTION ( 'NONE',  ( 7.125109674141484573E-05, -0.9999848031710252272, 0.005512562950851785694 ) ) ;
#2231=VECTOR ( 'NONE', #10553, 1000.000000000000000 ) ;
#2243=CARTESIAN_POINT ( 'NONE',  ( 18.63479515211382420, 189.4186551486400845, -105.7525706519799797 ) ) ;
#2252=ORIENTED_EDGE ( 'NONE', *, *, #17979, .F. ) ;
#2256=CARTESIAN_POINT ( 'NONE',  ( -48.56578001921132426, 94.99786382055523859, -43.46314047150291060 ) ) ;
#2270=SHAPE_REPRESENTATION ( 'Movable Vise Jaw Block', ( #6292 ), #7747 ) ;
#2274=EDGE_LOOP ( 'NONE', ( #14704, #22602, #20055, #8156, #2494 ) ) ;
#2281=AXIS2_PLACEMENT_3D ( 'NONE', #6633, #2956, #15282 ) ;
#2291=DIRECTION ( 'NONE',  ( -0.01292394549866743465, -0.005513023399721021615, -0.9999012842304692006 ) ) ;
#2298=AXIS2_PLACEMENT_3D ( 'NONE', #3309, #5253, #17221 ) ;
#2310=FACE_OUTER_BOUND ( 'NONE', #11461, .T. ) ;
#2312=ORIENTED_EDGE ( 'NONE', *, *, #2553, .T. ) ;
#2320=ORIENTED_EDGE ( 'NONE', *, *, #11242, .F. ) ;
#2322=CARTESIAN_POINT ( 'NONE',  ( 50.15804862953017818, 189.5999982876588774, -73.26417670677410854 ) ) ;
#2326=DIRECTION ( 'NONE',  ( 0.9999164797902017066, 6.884683795282953926E-18, -0.01292414190464158570 ) ) ;
#2330=CARTESIAN_POINT ( 'NONE',  ( 40.15436401027564273, 105.7502092278853496, 91.83706941573649374 ) ) ;
#2342=CARTESIAN_POINT ( 'NONE',  ( 39.45263645499988314, 96.15465585523027414, -42.60697859377187058 ) ) ;
#2345=CARTESIAN_POINT ( 'NONE',  ( -37.41279527276211070, 95.93415318215261323, 85.10526972611022245 ) ) ;
#2346=DIRECTION ( 'NONE',  ( -0.01292394549866739996, -0.005513023399721131770, -0.9999012842304692006 ) ) ;
#2350=CARTESIAN_POINT ( 'NONE',  ( 64.42259306105445660, 139.7551263635816952, -45.17031240767400391 ) ) ;
#2358=DIRECTION ( 'NONE',  ( -0.01292394549866739996, -0.005513023399721131770, -0.9999012842304692006 ) ) ;
#2361=CIRCLE ( 'NONE', #15225, 75.00000000000002842 ) ;
#2368=AXIS2_PLACEMENT_3D ( 'NONE', #19561, #16036, #5422 ) ;
#2370=EDGE_CURVE ( 'NONE', #19195, #5966, #3250, .T. ) ;
#2377=FACE_OUTER_BOUND ( 'NONE', #15801, .T. ) ;
#2380=CARTESIAN_POINT ( 'NONE',  ( -39.15186314103204523, 101.1708071963161615, 65.87724253366035043 ) ) ;
#2393=CARTESIAN_POINT ( 'NONE',  ( -53.19758388046658126, 169.4872888238259634, -92.31876405439228961 ) ) ;
#2396=VERTEX_POINT ( 'NONE', #22170 ) ;
#2397=CARTESIAN_POINT ( 'NONE',  ( -46.77184957787964237, 141.3748088146942621, 250.0790257996952164 ) ) ;
#2402=ORIENTED_EDGE ( 'NONE', *, *, #18477, .F. ) ;
#2407=ORIENTED_EDGE ( 'NONE', *, *, #21818, .T. ) ;
#2408=CARTESIAN_POINT ( 'NONE',  ( 51.12450654134402583, 113.4816418268618037, -44.85357105984766690 ) ) ;
#2415=VERTEX_POINT ( 'NONE', #242 ) ;
#2420=CARTESIAN_POINT ( 'NONE',  ( 41.18571742869637120, 107.5562382960386856, 71.06825843561573208 ) ) ;
#2435=EDGE_LOOP ( 'NONE', ( #21478, #4282, #13507, #21390 ) ) ;
#2437=CARTESIAN_POINT ( 'NONE',  ( 49.04937187465694137, 189.5912358487612437, -74.83936258294382071 ) ) ;
#2441=CARTESIAN_POINT ( 'NONE',  ( -41.07974036897499559, 106.8060942374655156, 71.47017004102838200 ) ) ;
#2444=ORIENTED_EDGE ( 'NONE', *, *, #5205, .T. ) ;
#2452=CARTESIAN_POINT ( 'NONE',  ( 39.88384264372077581, 95.41938954526496275, -43.87626177154204044 ) ) ;
#2463=B_SPLINE_CURVE_WITH_KNOTS ( 'NONE', 3,
 ( #19881, #14417, #19761, #9559, #494, #21491, #4148, #12784, #11059, #18083, #2330, #16372, #9433, #16475, #19032, #15396 ),
 .UNSPECIFIED., .F., .F.,
 ( 4, 2, 2, 2, 2, 2, 2, 4 ),
 ( 0.000000000000000000, 0.0008650928527149638831, 0.001297639279072451083, 0.001730185705429938391, 0.002162732131787425700, 0.002595278558144913008, 0.003027824984502400316, 0.003460371410859887625 ),
 .UNSPECIFIED. ) ;
#2465=CARTESIAN_POINT ( 'NONE',  ( -52.96495286149056625, 169.5865232450209703, -74.32054093824388019 ) ) ;
#2470=CARTESIAN_POINT ( 'NONE',  ( 47.42524840967396216, 108.3817487785542824, -44.77763872393808953 ) ) ;
#2472=CARTESIAN_POINT ( 'NONE',  ( 40.93051939605364709, 108.3240682923980245, 71.73403676058168799 ) ) ;
#2473=EDGE_CURVE ( 'NONE', #850, #163, #22598, .T. ) ;
#2474=ORIENTED_EDGE ( 'NONE', *, *, #8003, .F. ) ;
#2479=LINE ( 'NONE', #16638, #8903 ) ;
#2480=VERTEX_POINT ( 'NONE', #12323 ) ;
#2484=CARTESIAN_POINT ( 'NONE',  ( -39.85978252003874189, 107.1149823552814269, 71.72844665203564318 ) ) ;
#2486=ADVANCED_FACE ( 'NONE', ( #12422 ), #14159, .T. ) ;
#2491=VERTEX_POINT ( 'NONE', #13914 ) ;
#2494=ORIENTED_EDGE ( 'NONE', *, *, #1966, .T. ) ;
#2499=EDGE_LOOP ( 'NONE', ( #16336, #18855, #5489, #8445, #12361, #7673 ) ) ;
#2510=FACE_OUTER_BOUND ( 'NONE', #6210, .T. ) ;
#2512=VERTEX_POINT ( 'NONE', #3459 ) ;
#2513=ORIENTED_EDGE ( 'NONE', *, *, #7647, .F. ) ;
#2519=AXIS2_PLACEMENT_3D ( 'NONE', #5317, #3493, #9099 ) ;
#2520=EDGE_CURVE ( 'NONE', #11415, #7916, #1737, .T. ) ;
#2525=CARTESIAN_POINT ( 'NONE',  ( 42.65070472731144235, 106.8158425704275771, 70.39662431911894203 ) ) ;
#2531=AXIS2_PLACEMENT_3D ( 'NONE', #17874, #3379, #11408 ) ;
#2533=CARTESIAN_POINT ( 'NONE',  ( 51.99565694909048830, 170.0000000000000284, -0.6720553790413839046 ) ) ;
#2534=CARTESIAN_POINT ( 'NONE',  ( -52.09476476361207631, 111.8005892369645551, -46.74040084276866480 ) ) ;
#2536=CARTESIAN_POINT ( 'NONE',  ( -48.59517321819919289, 144.7440243326373945, -45.73723683152278596 ) ) ;
#2540=CARTESIAN_POINT ( 'NONE',  ( -49.99582398951009310, 170.0000000000008242, 0.6462070952329234119 ) ) ;
#2548=CARTESIAN_POINT ( 'NONE',  ( -38.81723620139342046, 107.2561214313139999, 91.76669763212666453 ) ) ;
#2553=EDGE_CURVE ( 'NONE', #13904, #956, #6408, .T. ) ;
#2555=ORIENTED_EDGE ( 'NONE', *, *, #21257, .F. ) ;
#2558=ORIENTED_EDGE ( 'NONE', *, *, #5122, .T. ) ;
#2562=CIRCLE ( 'NONE', #19035, 9.921742784567044282 ) ;
#2565=CARTESIAN_POINT ( 'NONE',  ( -36.94622273008864966, 105.5072037373731888, 92.66402702562507443 ) ) ;
#2570=CARTESIAN_POINT ( 'NONE',  ( -38.65774199683229284, 93.42233106614874316, 84.97233930033243610 ) ) ;
#2571=ORIENTED_EDGE ( 'NONE', *, *, #17694, .T. ) ;
#2577=DIRECTION ( 'NONE',  ( -0.01292394549866740169, -0.005513023399719847208, -0.9999012842304693116 ) ) ;
#2578=ORIENTED_EDGE ( 'NONE', *, *, #17644, .F. ) ;
#2592=DIRECTION ( 'NONE',  ( 7.125109674161246868E-05, -0.9999848031710252272, 0.005512562950850154186 ) ) ;
#2596=DIRECTION ( 'NONE',  ( -0.9999164797902017066, -6.965998958219367529E-18, 0.01292414190464157182 ) ) ;
#2599=AXIS2_PLACEMENT_3D ( 'NONE', #22430, #3046, #15141 ) ;
#2603=DIRECTION ( 'NONE',  ( -0.01292394549866740690, -0.005513023399721241925, -0.9999012842304693116 ) ) ;
#2605=CARTESIAN_POINT ( 'NONE',  ( 41.20321018459106455, 119.3672327899910073, 247.5807606757190911 ) ) ;
#2610=CARTESIAN_POINT ( 'NONE',  ( 48.56730888123496470, 169.3906321239456361, -111.1677263521955155 ) ) ;
#2622=AXIS2_PLACEMENT_3D ( 'NONE', #9816, #11654, #18649 ) ;
#2634=CARTESIAN_POINT ( 'NONE',  ( -37.91542670742843057, 96.08856300483259361, 84.97300045992372475 ) ) ;
#2637=ORIENTED_EDGE ( 'NONE', *, *, #20551, .T. ) ;
#2653=CARTESIAN_POINT ( 'NONE',  ( -50.37006368079059371, 112.6452800717682408, -43.53711992947328469 ) ) ;
#2656=LINE ( 'NONE', #9774, #9230 ) ;
#2669=CARTESIAN_POINT ( 'NONE',  ( -10.85567112094788200, 105.6999953372425409, 127.2994028633183063 ) ) ;
#2673=VERTEX_POINT ( 'NONE', #11602 ) ;
#2685=ORIENTED_EDGE ( 'NONE', *, *, #19241, .F. ) ;
#2698=DIRECTION ( 'NONE',  ( -7.125109674243555432E-05, 0.9999848031710253382, -0.005512562950850175003 ) ) ;
#2701=VECTOR ( 'NONE', #8952, 999.9999999999998863 ) ;
#2708=CARTESIAN_POINT ( 'NONE',  ( 41.59766263983357248, 107.1788419875362877, 70.73196411567400332 ) ) ;
#2719=VERTEX_POINT ( 'NONE', #18822 ) ;
#2740=CARTESIAN_POINT ( 'NONE',  ( -10.85567112094788200, 105.6999953372425409, 127.2994028633183063 ) ) ;
#2743=AXIS2_PLACEMENT_3D ( 'NONE', #5360, #10324, #14558 ) ;
#2745=CARTESIAN_POINT ( 'NONE',  ( -38.79751061739447948, 129.3639651298425406, 248.0419808514072315 ) ) ;
#2746=VERTEX_POINT ( 'NONE', #16891 ) ;
#2764=CARTESIAN_POINT ( 'NONE',  ( -52.45527812472808193, 109.9911275598175280, -43.49553422157452331 ) ) ;
#2765=CARTESIAN_POINT ( 'NONE',  ( -49.99582398951010731, 170.0000000000000284, 0.6462070952320568828 ) ) ;
#2772=LINE ( 'NONE', #8163, #4173 ) ;
#2773=VERTEX_POINT ( 'NONE', #16681 ) ;
#2778=CARTESIAN_POINT ( 'NONE',  ( -38.92003986412552052, 97.39926864640099780, 83.81297216957182172 ) ) ;
#2780=EDGE_CURVE ( 'NONE', #13067, #2773, #20502, .T. ) ;
#2787=DIRECTION ( 'NONE',  ( 0.9999164797902017066, 6.965998958219365988E-18, -0.01292414190464157356 ) ) ;
#2793=VERTEX_POINT ( 'NONE', #18700 ) ;
#2807=EDGE_CURVE ( 'NONE', #13285, #8542, #5246, .T. ) ;
#2810=CARTESIAN_POINT ( 'NONE',  ( 49.99582398951009310, 170.0000000000008242, -0.6462070952312342076 ) ) ;
#2824=CARTESIAN_POINT ( 'NONE',  ( 41.99649215118846968, 170.0000000000000284, -0.5428139599949681759 ) ) ;
#2835=ADVANCED_FACE ( 'NONE', ( #11945 ), #19036, .T. ) ;
#2839=EDGE_LOOP ( 'NONE', ( #21238, #1221, #2402, #11138 ) ) ;
#2844=VERTEX_POINT ( 'NONE', #19272 ) ;
#2850=ORIENTED_EDGE ( 'NONE', *, *, #15533, .F. ) ;
#2852=EDGE_CURVE ( 'NONE', #1571, #21136, #15624, .T. ) ;
#2864=CARTESIAN_POINT ( 'NONE',  ( -51.07137216368364818, 109.3042685136236685, -43.50963446871423201 ) ) ;
#2870=AXIS2_PLACEMENT_3D ( 'NONE', #19684, #17787, #2025 ) ;
#2871=CARTESIAN_POINT ( 'NONE',  ( 44.03028354117878251, 168.0879242961143518, -75.31593853751020617 ) ) ;
#2879=LINE ( 'NONE', #6666, #10748 ) ;
#2883=DIRECTION ( 'NONE',  ( -0.01292394549866740169, -0.005513023399721131770, -0.9999012842304693116 ) ) ;
#2893=DIRECTION ( 'NONE',  ( 0.01292394549866695240, 0.005513023399718316314, 0.9999012842304693116 ) ) ;
#2898=CIRCLE ( 'NONE', #17962, 1.999999999999999778 ) ;
#2902=ORIENTED_EDGE ( 'NONE', *, *, #11528, .F. ) ;
#2905=CARTESIAN_POINT ( 'NONE',  ( -46.79684245571608869, 129.3639651298425406, 248.1453739866443868 ) ) ;
#2906=CARTESIAN_POINT ( 'NONE',  ( -49.99582398951010731, 170.0000000000000284, 0.6462070952320568828 ) ) ;
#2908=CARTESIAN_POINT ( 'NONE',  ( -40.67014407421521582, 94.95224308429735061, 83.45134616373267988 ) ) ;
#2913=CARTESIAN_POINT ( 'NONE',  ( -49.22153082712133454, 106.9149828242082947, 60.55180848632685553 ) ) ;
#2915=EDGE_LOOP ( 'NONE', ( #19963, #6877, #703, #3281 ) ) ;
#2918=ORIENTED_EDGE ( 'NONE', *, *, #10272, .F. ) ;
#2921=ORIENTED_EDGE ( 'NONE', *, *, #4620, .T. ) ;
#2922=LINE ( 'NONE', #884, #17279 ) ;
#2940=ORIENTED_EDGE ( 'NONE', *, *, #11242, .T. ) ;
#2956=DIRECTION ( 'NONE',  ( 0.9999164797902017066, 6.965998958219365988E-18, -0.01292414190464157356 ) ) ;
#2963=ORIENTED_EDGE ( 'NONE', *, *, #5122, .F. ) ;
#2964=CARTESIAN_POINT ( 'NONE',  ( 45.22160658036679592, 125.3750519639578727, 248.9782057516816849 ) ) ;
#2971=DIRECTION ( 'NONE',  ( -0.01292394549866740169, -0.005513023399721021615, -0.9999012842304692006 ) ) ;
#2973=DIRECTION ( 'NONE',  ( 0.9999164797902017066, 6.965998958219367529E-18, -0.01292414190464157182 ) ) ;
#2977=CARTESIAN_POINT ( 'NONE',  ( -52.60896573992756942, 111.9218655255082524, -46.77848885693063608 ) ) ;
#2979=DIRECTION ( 'NONE',  ( 0.01292394549866738782, 0.005513023399721131770, 0.9999012842304692006 ) ) ;
#2988=CARTESIAN_POINT ( 'NONE',  ( -50.56880203129856000, 139.7551263635817236, -43.68402316449832057 ) ) ;
#2991=DIRECTION ( 'NONE',  ( 0.9999164797902015955, 6.965998958219364448E-18, -0.01292414190464157182 ) ) ;
#2996=DIRECTION ( 'NONE',  ( 0.9999164797902015955, 6.965998958219364448E-18, -0.01292414190464157182 ) ) ;
#2998=ORIENTED_EDGE ( 'NONE', *, *, #8247, .F. ) ;
#2999=AXIS2_PLACEMENT_3D ( 'NONE', #12428, #14512, #8849 ) ;
#3003=ORIENTED_EDGE ( 'NONE', *, *, #17644, .T. ) ;
#3007=DIRECTION ( 'NONE',  ( 0.01292394549866743812, 0.005513023399720639109, 0.9999012842304693116 ) ) ;
#3014=AXIS2_PLACEMENT_3D ( 'NONE', #645, #9128, #16179 ) ;
#3019=CARTESIAN_POINT ( 'NONE',  ( -20.57109388430227881, 136.7551719540686008, -44.05520973278501629 ) ) ;
#3021=DIRECTION ( 'NONE',  ( 0.01292394549868127775, 0.005513023399721131770, 0.9999012842304690896 ) ) ;
#3028=EDGE_CURVE ( 'NONE', #10034, #2793, #9147, .T. ) ;
#3029=EDGE_LOOP ( 'NONE', ( #20083, #8455, #1204, #1954 ) ) ;
#3038=DIRECTION ( 'NONE',  ( 0.009371490965938892789, 0.6886276452575282869, 0.7250545781830131098 ) ) ;
#3046=DIRECTION ( 'NONE',  ( 0.9999164797902015955, 6.965998958219364448E-18, -0.01292414190464157182 ) ) ;
#3051=CIRCLE ( 'NONE', #21734, 95.00000000000001421 ) ;
#3053=CARTESIAN_POINT ( 'NONE',  ( -39.48280323120003032, 107.3915498679189682, 71.96693194386834591 ) ) ;
#3054=VERTEX_POINT ( 'NONE', #19146 ) ;
#3055=ADVANCED_FACE ( 'NONE', ( #3421 ), #10543, .F. ) ;
#3069=CARTESIAN_POINT ( 'NONE',  ( 39.43544423852503655, 124.9314917220301737, -43.93710795200372843 ) ) ;
#3074=ORIENTED_EDGE ( 'NONE', *, *, #22228, .T. ) ;
#3077=AXIS2_PLACEMENT_3D ( 'NONE', #16306, #5582, #16188 ) ;
#3081=ORIENTED_EDGE ( 'NONE', *, *, #15743, .F. ) ;
#3083=CARTESIAN_POINT ( 'NONE',  ( 50.91257692374890809, 106.8061942917681790, 70.28123811582710800 ) ) ;
#3091=EDGE_LOOP ( 'NONE', ( #13209, #20791, #10498, #3830 ) ) ;
#3097=DIRECTION ( 'NONE',  ( 7.125109674161246868E-05, -0.9999848031710252272, 0.005512562950850154186 ) ) ;
#3102=CARTESIAN_POINT ( 'NONE',  ( 0.000000000000000000, 0.000000000000000000, 0.000000000000000000 ) ) ;
#3119=EDGE_LOOP ( 'NONE', ( #3878, #1092, #5398, #5843 ) ) ;
#3125=CARTESIAN_POINT ( 'NONE',  ( 50.24995405803858262, 113.2674379272951910, -44.84108624765922713 ) ) ;
#3127=CARTESIAN_POINT ( 'NONE',  ( -51.86045928498519686, 189.4905222308084660, -91.80463846584517285 ) ) ;
#3130=LINE ( 'NONE', #9808, #9170 ) ;
#3145=CARTESIAN_POINT ( 'NONE',  ( -49.34917620029669649, 107.4660479794951584, 70.81942874090999851 ) ) ;
#3155=CARTESIAN_POINT ( 'NONE',  ( -52.66211423087264620, 189.6011917897851333, -71.71870077557677803 ) ) ;
#3158=LINE ( 'NONE', #4757, #9574 ) ;
#3163=VERTEX_POINT ( 'NONE', #16345 ) ;
#3174=ORIENTED_EDGE ( 'NONE', *, *, #22256, .F. ) ;
#3179=DIRECTION ( 'NONE',  ( -0.9999164797902015955, -6.965998958219364448E-18, 0.01292414190464157182 ) ) ;
#3187=DIRECTION ( 'NONE',  ( 0.01292394549866695240, 0.005513023399718316314, 0.9999012842304693116 ) ) ;
#3192=CARTESIAN_POINT ( 'NONE',  ( -64.07781940414963628, 106.8060942374655156, 71.76742530483514315 ) ) ;
#3204=CARTESIAN_POINT ( 'NONE',  ( 53.21979840114054383, 141.3748088146942621, 248.7866116092309881 ) ) ;
#3209=VECTOR ( 'NONE', #7295, 1000.000000000000114 ) ;
#3210=ORIENTED_EDGE ( 'NONE', *, *, #9343, .T. ) ;
#3212=CARTESIAN_POINT ( 'NONE',  ( 14.14167086503323034, 113.6998737626107641, 126.9321988120954643 ) ) ;
#3218=VERTEX_POINT ( 'NONE', #12658 ) ;
#3221=LINE ( 'NONE', #5055, #9631 ) ;
#3228=ORIENTED_EDGE ( 'NONE', *, *, #13506, .F. ) ;
#3230=DIRECTION ( 'NONE',  ( 0.9999164797902017066, 6.965998958219365988E-18, -0.01292414190464157356 ) ) ;
#3231=DIRECTION ( 'NONE',  ( 0.01096700916508639573, -0.5290868411612598132, 0.8484968115555726609 ) ) ;
#3233=AXIS2_PLACEMENT_3D ( 'NONE', #17889, #9120, #2123 ) ;
#3245=VECTOR ( 'NONE', #11608, 1000.000000000000000 ) ;
#3248=CARTESIAN_POINT ( 'NONE',  ( -49.09967157776827662, 108.0238286078847523, 69.97982874036236467 ) ) ;
#3250=CIRCLE ( 'NONE', #12059, 2.000000000000001332 ) ;
#3251=CARTESIAN_POINT ( 'NONE',  ( 50.79397376011281295, 189.4876967392748384, -93.64401692289283119 ) ) ;
#3253=CARTESIAN_POINT ( 'NONE',  ( -49.99582398951010731, 170.0000000000000284, 0.6462070952320568828 ) ) ;
#3255=DIRECTION ( 'NONE',  ( -0.003413786507416180071, 0.9644842718275419280, -0.2641182225045783927 ) ) ;
#3256=FACE_OUTER_BOUND ( 'NONE', #22115, .T. ) ;
#3258=CARTESIAN_POINT ( 'NONE',  ( 51.07319921393754214, 94.45452722259994971, 82.70828171889884572 ) ) ;
#3274=CARTESIAN_POINT ( 'NONE',  ( 44.03052579490771024, 164.6879759653328961, -75.29719582347730977 ) ) ;
#3281=ORIENTED_EDGE ( 'NONE', *, *, #13013, .T. ) ;
#3285=ORIENTED_EDGE ( 'NONE', *, *, #2807, .F. ) ;
#3287=CIRCLE ( 'NONE', #16542, 2.009999999999995346 ) ;
#3289=ORIENTED_EDGE ( 'NONE', *, *, #5069, .F. ) ;
#3295=AXIS2_PLACEMENT_3D ( 'NONE', #12700, #16615, #13152 ) ;
#3301=DIRECTION ( 'NONE',  ( 7.125109674159586684E-05, -0.9999848031710252272, 0.005512562950848869624 ) ) ;
#3306=CARTESIAN_POINT ( 'NONE',  ( 19.85645766388354971, -0.1201756712316815051, -11.23484659157417376 ) ) ;
#3307=ORIENTED_EDGE ( 'NONE', *, *, #8778, .T. ) ;
#3309=CARTESIAN_POINT ( 'NONE',  ( 40.84145524218410372, 101.1708071963161615, 64.84331118128903881 ) ) ;
#3311=CARTESIAN_POINT ( 'NONE',  ( 64.42223680557074772, 144.7550503794368524, -45.19787522242825162 ) ) ;
#3316=ORIENTED_EDGE ( 'NONE', *, *, #19103, .T. ) ;
#3318=CARTESIAN_POINT ( 'NONE',  ( -49.94445001183338917, 112.2316389946799120, -43.54034044231270428 ) ) ;
#3319=VECTOR ( 'NONE', #11175, 1000.000000000000000 ) ;
#3322=CARTESIAN_POINT ( 'NONE',  ( 50.66019270109019601, 111.6821163282932190, -48.02485136456311210 ) ) ;
#3327=DIRECTION ( 'NONE',  ( -7.125109674161246868E-05, 0.9999848031710252272, -0.005512562950850154186 ) ) ;
#3331=CARTESIAN_POINT ( 'NONE',  ( -40.54592687530145412, 169.7656965055118974, -41.97883890360929371 ) ) ;
#3333=AXIS2_PLACEMENT_3D ( 'NONE', #10042, #14691, #6583 ) ;
#3347=ORIENTED_EDGE ( 'NONE', *, *, #16474, .T. ) ;
#3352=CARTESIAN_POINT ( 'NONE',  ( 41.99649215118846968, 170.0000000000000284, -0.5428139599949681759 ) ) ;
#3353=ORIENTED_EDGE ( 'NONE', *, *, #20397, .T. ) ;
#3355=CARTESIAN_POINT ( 'NONE',  ( -19.99832959580404790, 170.0000000000008242, 0.2584828380936761705 ) ) ;
#3358=EDGE_CURVE ( 'NONE', #13022, #13585, #17113, .T. ) ;
#3370=ORIENTED_EDGE ( 'NONE', *, *, #17786, .F. ) ;
#3374=ADVANCED_FACE ( 'NONE', ( #19494 ), #22460, .F. ) ;
#3379=DIRECTION ( 'NONE',  ( 0.9999164797902017066, 6.965998958219365988E-18, -0.01292414190464157356 ) ) ;
#3382=CARTESIAN_POINT ( 'NONE',  ( 40.93051939605364709, 108.3240682923980245, 71.73403676058168799 ) ) ;
#3383=AXIS2_PLACEMENT_3D ( 'NONE', #19415, #9312, #11040 ) ;
#3395=CARTESIAN_POINT ( 'NONE',  ( 49.38251519867302619, 111.9218655255082382, -48.09675133120408219 ) ) ;
#3401=VECTOR ( 'NONE', #12889, 1000.000000000000114 ) ;
#3403=( BOUNDED_CURVE ( )  B_SPLINE_CURVE ( 3, ( #10190, #3069, #20636, #4891 ),
 .UNSPECIFIED., .F., .T. ) 
 B_SPLINE_CURVE_WITH_KNOTS ( ( 4, 4 ),
 ( 4.712388980384689674, 6.283185307179586232 ),
 .UNSPECIFIED. ) 
 CURVE ( )  GEOMETRIC_REPRESENTATION_ITEM ( )  RATIONAL_B_SPLINE_CURVE ( ( 1.000000000000000000, 0.8047378541243649375, 0.8047378541243649375, 1.000000000000000000 ) ) 
 REPRESENTATION_ITEM ( '' )  );
#3404=CIRCLE ( 'NONE', #6707, 2.000000000000005329 ) ;
#3421=FACE_OUTER_BOUND ( 'NONE', #11045, .T. ) ;
#3431=LINE ( 'NONE', #10328, #17717 ) ;
#3434=FACE_OUTER_BOUND ( 'NONE', #12563, .T. ) ;
#3436=FACE_OUTER_BOUND ( 'NONE', #18085, .T. ) ;
#3441=CARTESIAN_POINT ( 'NONE',  ( -50.37155587173380411, 112.6465223951286276, -43.53710749220883969 ) ) ;
#3444=CARTESIAN_POINT ( 'NONE',  ( 50.07407138682150816, 111.0341656543122184, -47.77903772492574319 ) ) ;
#3449=EDGE_CURVE ( 'NONE', #9196, #2793, #6061, .T. ) ;
#3459=CARTESIAN_POINT ( 'NONE',  ( 44.00388087554392769, 168.0766615966952884, -77.35866297318138152 ) ) ;
#3473=ORIENTED_EDGE ( 'NONE', *, *, #4996, .T. ) ;
#3475=FACE_OUTER_BOUND ( 'NONE', #13358, .T. ) ;
#3487=ORIENTED_EDGE ( 'NONE', *, *, #10058, .F. ) ;
#3489=UNCERTAINTY_MEASURE_WITH_UNIT (LENGTH_MEASURE( 1.000000000000000082E-05 ), #4259, 'distance_accuracy_value', 'NONE');
#3493=DIRECTION ( 'NONE',  ( 0.9999164797902015955, 6.965998958219364448E-18, -0.01292414190464157182 ) ) ;
#3504=ORIENTED_EDGE ( 'NONE', *, *, #4006, .T. ) ;
#3505=DIRECTION ( 'NONE',  ( -0.01246513159389404414, -0.2641402835564772844, -0.9644037178988117409 ) ) ;
#3524=ADVANCED_FACE ( 'NONE', ( #13091, #7440, #9150 ), #3877, .T. ) ;
#3526=EDGE_CURVE ( 'NONE', #5966, #15010, #21445, .T. ) ;
#3531=PLANE ( 'NONE',  #9914 ) ;
#3533=LINE ( 'NONE', #17008, #13609 ) ;
#3538=DIRECTION ( 'NONE',  ( 7.125109674161246868E-05, -0.9999848031710253382, 0.005512562950850155054 ) ) ;
#3539=CARTESIAN_POINT ( 'NONE',  ( -66.42308629463825298, 169.3906321239456361, -109.6814500331617381 ) ) ;
#3540=CARTESIAN_POINT ( 'NONE',  ( -50.60480870902609496, 108.7763774210405501, -45.65653423414172352 ) ) ;
#3551=CARTESIAN_POINT ( 'NONE',  ( 50.28732129150708374, 111.3287588133958081, -47.88997685343035471 ) ) ;
#3562=ORIENTED_EDGE ( 'NONE', *, *, #1372, .F. ) ;
#3566=ORIENTED_EDGE ( 'NONE', *, *, #7415, .T. ) ;
#3572=AXIS2_PLACEMENT_3D ( 'NONE', #20438, #17237, #4693 ) ;
#3574=ORIENTED_EDGE ( 'NONE', *, *, #11205, .F. ) ;
#3576=VERTEX_POINT ( 'NONE', #21541 ) ;
#3591=ORIENTED_EDGE ( 'NONE', *, *, #20551, .F. ) ;
#3595=ORIENTED_EDGE ( 'NONE', *, *, #13094, .T. ) ;
#3598=FACE_OUTER_BOUND ( 'NONE', #8961, .T. ) ;
#3600=VECTOR ( 'NONE', #15211, 1000.000000000000000 ) ;
#3602=CARTESIAN_POINT ( 'NONE',  ( -38.85108570016819129, 97.00796024230733394, 84.16132632256042712 ) ) ;
#3611=LINE ( 'NONE', #3944, #10665 ) ;
#3615=AXIS2_PLACEMENT_3D ( 'NONE', #3352, #6792, #1313 ) ;
#3628=VECTOR ( 'NONE', #4347, 1000.000000000000114 ) ;
#3643=ORIENTED_EDGE ( 'NONE', *, *, #6245, .F. ) ;
#3655=CARTESIAN_POINT ( 'NONE',  ( 53.22065341430143803, 129.3749911766419700, 248.8527623646411939 ) ) ;
#3656=ORIENTED_EDGE ( 'NONE', *, *, #9205, .F. ) ;
#3657=CARTESIAN_POINT ( 'NONE',  ( -50.99271059757531788, 113.0670368246753554, -43.53139746460606574 ) ) ;
#3667=LINE ( 'NONE', #582, #19624 ) ;
#3688=DIRECTION ( 'NONE',  ( 0.9999164797902015955, 6.965998958219364448E-18, -0.01292414190464157182 ) ) ;
#3695=AXIS2_PLACEMENT_3D ( 'NONE', #21587, #2326, #11054 ) ;
#3706=CARTESIAN_POINT ( 'NONE',  ( 19.42556530730579567, 136.7551719540686008, -44.57217540897067920 ) ) ;
#3720=AXIS2_PLACEMENT_3D ( 'NONE', #12103, #3021, #13720 ) ;
#3729=CARTESIAN_POINT ( 'NONE',  ( 48.58946335778052372, 189.4003865961453812, -109.4536762928195230 ) ) ;
#3735=ORIENTED_EDGE ( 'NONE', *, *, #13178, .T. ) ;
#3737=AXIS2_PLACEMENT_3D ( 'NONE', #2536, #9665, #14739 ) ;
#3739=ADVANCED_FACE ( 'NONE', ( #22377 ), #6780, .T. ) ;
#3741=EDGE_CURVE ( 'NONE', #13237, #5372, #296, .T. ) ;
#3744=CARTESIAN_POINT ( 'NONE',  ( 14.19595143612763444, 113.7230284608895943, 131.1317842058634255 ) ) ;
#3759=EDGE_CURVE ( 'NONE', #21389, #17449, #679, .T. ) ;
#3762=EDGE_CURVE ( 'NONE', #21685, #9499, #11859, .T. ) ;
#3765=DIRECTION ( 'NONE',  ( 0.01292394549866740169, 0.005513023399720822990, 0.9999012842304693116 ) ) ;
#3770=CARTESIAN_POINT ( 'NONE',  ( -38.77166272639713185, 129.3749911766419700, 250.0417834198682101 ) ) ;
#3774=FACE_OUTER_BOUND ( 'NONE', #6813, .T. ) ;
#3779=CARTESIAN_POINT ( 'NONE',  ( -52.56676294784124792, 113.4816418249608034, -43.51333844217711544 ) ) ;
#3781=CARTESIAN_POINT ( 'NONE',  ( -49.12744300538584952, 95.04215844998273610, -43.53116934361613488 ) ) ;
#3794=VERTEX_POINT ( 'NONE', #1304 ) ;
#3810=LINE ( 'NONE', #19544, #8762 ) ;
#3824=DIRECTION ( 'NONE',  ( 0.01246513159389404414, 0.2641402835564772844, 0.9644037178988117409 ) ) ;
#3830=ORIENTED_EDGE ( 'NONE', *, *, #7238, .F. ) ;
#3842=ORIENTED_EDGE ( 'NONE', *, *, #8919, .F. ) ;
#3848=MECHANICAL_DESIGN_GEOMETRIC_PRESENTATION_REPRESENTATION('',(#6432),#20715);
#3851=ORIENTED_EDGE ( 'NONE', *, *, #11320, .F. ) ;
#3852=CARTESIAN_POINT ( 'NONE',  ( -66.32153322427998887, 169.4339520569534159, -101.8244805435235918 ) ) ;
#3854=EDGE_LOOP ( 'NONE', ( #15281, #11812, #16723 ) ) ;
#3858=CIRCLE ( 'NONE', #4941, 2.000000000000005773 ) ;
#3864=VERTEX_POINT ( 'NONE', #1250 ) ;
#3873=ORIENTED_EDGE ( 'NONE', *, *, #532, .F. ) ;
#3877=PLANE ( 'NONE',  #17995 ) ;
#3878=ORIENTED_EDGE ( 'NONE', *, *, #3762, .T. ) ;
#3881=EDGE_CURVE ( 'NONE', #20719, #7056, #6943, .T. ) ;
#3882=CARTESIAN_POINT ( 'NONE',  ( -42.56847267762256593, 125.7553391191873544, -43.71024041842355246 ) ) ;
#3887=ORIENTED_EDGE ( 'NONE', *, *, #18824, .T. ) ;
#3898=ORIENTED_EDGE ( 'NONE', *, *, #5677, .F. ) ;
#3907=CARTESIAN_POINT ( 'NONE',  ( -64.99457118636313169, 170.0000000000000284, 0.8400692238016805868 ) ) ;
#3919=EDGE_CURVE ( 'NONE', #5652, #22611, #12407, .T. ) ;
#3920=DIRECTION ( 'NONE',  ( 0.9999164797902017066, 6.965998958219367529E-18, -0.01292414190464157182 ) ) ;
#3921=CARTESIAN_POINT ( 'NONE',  ( 65.91132296857659867, 106.8060942374655156, 70.08728685723174578 ) ) ;
#3938=CARTESIAN_POINT ( 'NONE',  ( -10.80367058494921118, 137.7226637369942068, 131.3225862426590709 ) ) ;
#3944=CARTESIAN_POINT ( 'NONE',  ( -35.41655530694463749, 106.0996895337223407, 200.1218115885957332 ) ) ;
#3950=DIRECTION ( 'NONE',  ( -0.01292394549866739996, -0.005513023399721131770, -0.9999012842304692006 ) ) ;
#3956=FACE_OUTER_BOUND ( 'NONE', #2161, .T. ) ;
#3960=LINE ( 'NONE', #4080, #21766 ) ;
#3961=CARTESIAN_POINT ( 'NONE',  ( 51.90570505437388249, 106.9898499841750521, 70.07644525255086876 ) ) ;
#3969=DIRECTION ( 'NONE',  ( -0.009088227368120585167, -0.7109943316365089361, -0.7031390079522393810 ) ) ;
#3991=CARTESIAN_POINT ( 'NONE',  ( -42.01023468938293348, 95.04007470540923919, -43.47457758741172285 ) ) ;
#3997=VECTOR ( 'NONE', #13077, 1000.000000000000114 ) ;
#4006=EDGE_CURVE ( 'NONE', #21984, #22611, #14328, .T. ) ;
#4008=EDGE_CURVE ( 'NONE', #2673, #16531, #9469, .T. ) ;
#4017=CARTESIAN_POINT ( 'NONE',  ( 14.04531128256715888, 105.6586476617446380, 119.4770396839737714 ) ) ;
#4031=CARTESIAN_POINT ( 'NONE',  ( -50.76769345292276370, 109.8130285628466538, -46.02948977673421638 ) ) ;
#4037=VERTEX_POINT ( 'NONE', #11550 ) ;
#4047=CARTESIAN_POINT ( 'NONE',  ( 39.80634724086582565, 95.47920460943406340, -43.77198102653553491 ) ) ;
#4051=CARTESIAN_POINT ( 'NONE',  ( 39.99665919160806027, 170.0000000000000284, -0.5169656761856848970 ) ) ;
#4056=LINE ( 'NONE', #18547, #5507 ) ;
#4059=VERTEX_POINT ( 'NONE', #13797 ) ;
#4065=ORIENTED_EDGE ( 'NONE', *, *, #15984, .F. ) ;
#4069=LINE ( 'NONE', #11098, #16202 ) ;
#4073=AXIS2_PLACEMENT_3D ( 'NONE', #2669, #21922, #7834 ) ;
#4080=CARTESIAN_POINT ( 'NONE',  ( -36.79753515562058652, 127.3639955235004777, 248.0271576934996745 ) ) ;
#4090=DIRECTION ( 'NONE',  ( -0.9999164797902017066, -6.965998958219365988E-18, 0.01292414190464157356 ) ) ;
#4093=ORIENTED_EDGE ( 'NONE', *, *, #10359, .T. ) ;
#4097=AXIS2_PLACEMENT_3D ( 'NONE', #21829, #18743, #3007 ) ;
#4101=AXIS2_PLACEMENT_3D ( 'NONE', #10906, #16100, #2291 ) ;
#4124=CARTESIAN_POINT ( 'NONE',  ( -64.99457118636311748, 170.0000000000008242, 0.8400692238025471159 ) ) ;
#4128=CARTESIAN_POINT ( 'NONE',  ( 40.58037928852487397, 106.1692389898096280, 199.3935091201308296 ) ) ;
#4129=( BOUNDED_SURFACE ( )  B_SPLINE_SURFACE ( 3, 2, ( 
 ( #1830, #6997, #6876 ),
 ( #20545, #15417, #8601 ),
 ( #17127, #14023, #8701 ),
 ( #21010, #6659, #13795 ),
 ( #17232, #20778, #5263 ),
 ( #15752, #11849, #12308 ),
 ( #1502, #19169, #5032 ),
 ( #8825, #6547, #12187 ),
 ( #3444, #13687, #10119 ),
 ( #3551, #18839, #20669 ),
 ( #10226, #12067, #4928 ),
 ( #3322, #1393, #15873 ),
 ( #10345, #11960, #10454 ),
 ( #19286, #18941, #13899 ),
 ( #20891, #10565, #2408 ),
 ( #9288, #19398, #17928 ) ),
 .UNSPECIFIED., .F., .F., .T. ) 
 B_SPLINE_SURFACE_WITH_KNOTS ( ( 4, 2, 2, 2, 2, 2, 2, 4 ),
 ( 3, 3 ),
 ( 0.003676974186938495454, 0.005450118764002107562, 0.006336691052533913182, 0.007223263341065719670, 0.008109835629597526158, 0.008996407918129330911, 0.009882980206661137398, 0.01076955249519294389 ),
 ( 0.000000000000000000, 1.000000000000000000 ),
 .UNSPECIFIED. ) 
 GEOMETRIC_REPRESENTATION_ITEM ( )  RATIONAL_B_SPLINE_SURFACE ( (
 ( 1.000000000000000000, 0.7071067811865460184, 1.000000000000000000),
 ( 1.000000000000000000, 0.6815104794066817462, 1.000000000000000000),
 ( 1.000000000000000000, 0.6547843716139309933, 1.000000000000000000),
 ( 1.000000000000000000, 0.6123586760872794521, 1.000000000000000000),
 ( 1.000000000000000000, 0.5978640991518743286, 1.000000000000000000),
 ( 1.000000000000000000, 0.5691342003131903970, 1.000000000000000000),
 ( 1.000000000000000000, 0.5547710840782603681, 1.000000000000000000),
 ( 1.000000000000000000, 0.5262790914882317095, 1.000000000000000000),
 ( 1.000000000000000000, 0.5119733473728251827, 1.000000000000000000),
 ( 1.000000000000000000, 0.4852625026393655450, 1.000000000000000000),
 ( 1.000000000000000000, 0.4728155099288974816, 1.000000000000000000),
 ( 1.000000000000000000, 0.4509953647258624909, 1.000000000000000000),
 ( 1.000000000000000000, 0.4419745220849347622, 1.000000000000000000),
 ( 1.000000000000000000, 0.4295065217292311499, 1.000000000000000000),
 ( 1.000000000000000000, 0.4259886279742503556, 1.000000000000000000),
 ( 1.000000000000000000, 0.4260362065776441831, 1.000000000000000000) ) ) 
 REPRESENTATION_ITEM ( '' )  SURFACE ( )  );
#4148=CARTESIAN_POINT ( 'NONE',  ( 40.76338182023881984, 106.2626885438830300, 92.18371853433509955 ) ) ;
#4163=CARTESIAN_POINT ( 'NONE',  ( -37.86293061927234049, 105.7860355035395230, 92.52957110793263951 ) ) ;
#4166=VECTOR ( 'NONE', #9917, 1000.000000000000000 ) ;
#4173=VECTOR ( 'NONE', #4589, 999.9999999999998863 ) ;
#4176=DIRECTION ( 'NONE',  ( 0.009188991635466048358, -0.7031977391749438810, 0.7109349492407661675 ) ) ;
#4184=ORIENTED_EDGE ( 'NONE', *, *, #864, .F. ) ;
#4185=CARTESIAN_POINT ( 'NONE',  ( 42.40290194442976457, 106.8542505984647164, 70.43401943659206665 ) ) ;
#4191=CARTESIAN_POINT ( 'NONE',  ( -37.41653076871853045, 108.0996591400643752, 200.1366347465033186 ) ) ;
#4197=AXIS2_PLACEMENT_3D ( 'NONE', #7495, #5872, #14526 ) ;
#4203=ORIENTED_EDGE ( 'NONE', *, *, #19091, .F. ) ;
#4215=CARTESIAN_POINT ( 'NONE',  ( -52.93127853433226448, 189.6011917897851333, -71.71522176735570042 ) ) ;
#4219=EDGE_LOOP ( 'NONE', ( #3643, #1404, #7748, #17028, #6097, #953, #20286, #4408, #15572 ) ) ;
#4223=ORIENTED_EDGE ( 'NONE', *, *, #7186, .F. ) ;
#4226=ORIENTED_EDGE ( 'NONE', *, *, #5069, .T. ) ;
#4236=CARTESIAN_POINT ( 'NONE',  ( 40.92823665025488822, 108.1171873888033872, 71.55742502417508888 ) ) ;
#4240=ORIENTED_EDGE ( 'NONE', *, *, #9720, .F. ) ;
#4243=CARTESIAN_POINT ( 'NONE',  ( -49.94283482827944454, 112.2298613550336057, -43.54035151778127499 ) ) ;
#4244=ORIENTED_EDGE ( 'NONE', *, *, #9205, .T. ) ;
#4251=ORIENTED_EDGE ( 'NONE', *, *, #5482, .F. ) ;
#4259=( LENGTH_UNIT ( ) NAMED_UNIT ( * ) SI_UNIT ( .MILLI., .METRE. ) );
#4260=CARTESIAN_POINT ( 'NONE',  ( -51.73689940103877660, 111.5659474609696105, -46.65855322351870171 ) ) ;
#4271=DIRECTION ( 'NONE',  ( 0.01292394549866738261, 0.005513023399722618428, 0.9999012842304692006 ) ) ;
#4277=AXIS2_PLACEMENT_3D ( 'NONE', #2540, #20330, #4804 ) ;
#4282=ORIENTED_EDGE ( 'NONE', *, *, #12026, .T. ) ;
#4284=DIRECTION ( 'NONE',  ( 0.01292394549866737220, 0.005513023399721000799, 0.9999012842304692006 ) ) ;
#4289=EDGE_LOOP ( 'NONE', ( #4240, #11007 ) ) ;
#4291=CARTESIAN_POINT ( 'NONE',  ( 42.03270152299423756, 106.9589643049704648, 70.53184856292322991 ) ) ;
#4292=EDGE_CURVE ( 'NONE', #16712, #4358, #14653, .T. ) ;
#4293=CARTESIAN_POINT ( 'NONE',  ( -45.96195738621045024, 164.6879759653328961, -74.13402305205957532 ) ) ;
#4309=CARTESIAN_POINT ( 'NONE',  ( 48.87608419539191829, 189.4960933113125634, -92.09608064579967390 ) ) ;
#4333=CARTESIAN_POINT ( 'NONE',  ( -40.55787414469111241, 124.9314917220301737, -42.90317659963240970 ) ) ;
#4345=ORIENTED_EDGE ( 'NONE', *, *, #21673, .F. ) ;
#4346=ORIENTED_EDGE ( 'NONE', *, *, #4609, .T. ) ;
#4347=DIRECTION ( 'NONE',  ( 0.01292394549866739996, 0.005513023399721131770, 0.9999012842304692006 ) ) ;
#4348=CARTESIAN_POINT ( 'NONE',  ( -52.68156204427607037, 109.2346208036755968, -43.48843840061612553 ) ) ;
#4353=DIRECTION ( 'NONE',  ( 0.01292394549866743812, 0.005513023399720639109, 0.9999012842304693116 ) ) ;
#4358=VERTEX_POINT ( 'NONE', #1417 ) ;
#4365=FACE_OUTER_BOUND ( 'NONE', #12111, .T. ) ;
#4372=ORIENTED_EDGE ( 'NONE', *, *, #710, .T. ) ;
#4408=ORIENTED_EDGE ( 'NONE', *, *, #14566, .T. ) ;
#4420=EDGE_CURVE ( 'NONE', #4059, #8542, #5805, .T. ) ;
#4427=VERTEX_POINT ( 'NONE', #11722 ) ;
#4430=ORIENTED_EDGE ( 'NONE', *, *, #8247, .T. ) ;
#4431=EDGE_CURVE ( 'NONE', #3218, #10523, #329, .T. ) ;
#4440=EDGE_CURVE ( 'NONE', #18473, #444, #9101, .T. ) ;
#4446=PLANE ( 'NONE',  #14227 ) ;
#4454=CARTESIAN_POINT ( 'NONE',  ( -38.71138566794451918, 96.73515328252067036, 84.40350015143866358 ) ) ;
#4455=DIRECTION ( 'NONE',  ( 0.01292394549867042185, 0.005513023399718316314, 0.9999012842304693116 ) ) ;
#4462=AXIS2_PLACEMENT_3D ( 'NONE', #1143, #1266, #4455 ) ;
#4468=CARTESIAN_POINT ( 'NONE',  ( -49.26081312276134838, 111.2483156817622927, -43.54375498084313278 ) ) ;
#4473=CARTESIAN_POINT ( 'NONE',  ( -48.67250884018650225, 109.5699351474431467, -43.54210507929712293 ) ) ;
#4496=AXIS2_PLACEMENT_3D ( 'NONE', #14594, #12742, #5819 ) ;
#4500=DIRECTION ( 'NONE',  ( 7.125109674161246868E-05, -0.9999848031710252272, 0.005512562950850154186 ) ) ;
#4502=DIRECTION ( 'NONE',  ( 7.125109674161246868E-05, -0.9999848031710253382, 0.005512562950850155054 ) ) ;
#4516=CIRCLE ( 'NONE', #1612, 2.000000000000001332 ) ;
#4525=CIRCLE ( 'NONE', #21716, 2.000000000000001332 ) ;
#4537=DIRECTION ( 'NONE',  ( -0.01292394549866740169, -0.005513023399721270548, -0.9999012842304692006 ) ) ;
#4543=CARTESIAN_POINT ( 'NONE',  ( 49.06618554817806910, 189.4933803444196201, -92.59067283796298398 ) ) ;
#4552=CARTESIAN_POINT ( 'NONE',  ( 51.07319921393754214, 94.45452722259994971, 82.70828171889884572 ) ) ;
#4560=ADVANCED_FACE ( 'NONE', ( #13226 ), #16454, .T. ) ;
#4562=ORIENTED_EDGE ( 'NONE', *, *, #12066, .F. ) ;
#4564=CARTESIAN_POINT ( 'NONE',  ( -38.13965839584966488, 96.20077325653890910, 84.87509721996781309 ) ) ;
#4570=VECTOR ( 'NONE', #264, 999.9999999999998863 ) ;
#4574=DIRECTION ( 'NONE',  ( -0.9999164797902015955, -6.965998958219364448E-18, 0.01292414190464157182 ) ) ;
#4577=SHAPE_DEFINITION_REPRESENTATION ( #12158, #2270 ) ;
#4581=CARTESIAN_POINT ( 'NONE',  ( -50.68129816702384005, 109.3835034331725780, -45.87488247214934489 ) ) ;
#4588=CYLINDRICAL_SURFACE ( 'NONE', #21872, 1.999999999999997780 ) ;
#4589=DIRECTION ( 'NONE',  ( 7.125109674161246868E-05, -0.9999848031710253382, 0.005512562950850155054 ) ) ;
#4598=ADVANCED_FACE ( 'NONE', ( #1034 ), #16501, .F. ) ;
#4605=TOROIDAL_SURFACE ( 'NONE', #1327, 93.00000000000000000, 2.000000000000000000 ) ;
#4609=EDGE_CURVE ( 'NONE', #18970, #7858, #18502, .T. ) ;
#4613=FACE_OUTER_BOUND ( 'NONE', #13813, .T. ) ;
#4620=EDGE_CURVE ( 'NONE', #848, #14385, #16569, .T. ) ;
#4633=ORIENTED_EDGE ( 'NONE', *, *, #18894, .T. ) ;
#4644=DIRECTION ( 'NONE',  ( -0.01292394549866737741, -0.005513023399721125699, -0.9999012842304693116 ) ) ;
#4648=ORIENTED_EDGE ( 'NONE', *, *, #9720, .T. ) ;
#4654=ORIENTED_EDGE ( 'NONE', *, *, #11950, .F. ) ;
#4658=CARTESIAN_POINT ( 'NONE',  ( -66.42677970909001317, 189.3893605493459233, -109.9672025422466959 ) ) ;
#4674=DIRECTION ( 'NONE',  ( -0.01292394549866739996, -0.005513023399721131770, -0.9999012842304692006 ) ) ;
#4682=LINE ( 'NONE', #11717, #10495 ) ;
#4687=ORIENTED_EDGE ( 'NONE', *, *, #18226, .T. ) ;
#4689=CARTESIAN_POINT ( 'NONE',  ( 41.19609277020862947, 125.3640259171584290, 247.0300997508393266 ) ) ;
#4693=DIRECTION ( 'NONE',  ( -0.01292394549866743465, -0.005513023399721021615, -0.9999012842304692006 ) ) ;
#4694=DIRECTION ( 'NONE',  ( -0.01292394549866739822, -0.005513023399721269681, -0.9999012842304692006 ) ) ;
#4701=CARTESIAN_POINT ( 'NONE',  ( -34.77142196148174946, 121.3072273804455250, 250.0345615839236757 ) ) ;
#4702=AXIS2_PLACEMENT_3D ( 'NONE', #17485, #19409, #20686 ) ;
#4703=ORIENTED_EDGE ( 'NONE', *, *, #7647, .T. ) ;
#4704=EDGE_CURVE ( 'NONE', #1703, #4037, #12814, .T. ) ;
#4718=CARTESIAN_POINT ( 'NONE',  ( -53.06372157685608215, 189.4876967392748952, -92.30163321429982659 ) ) ;
#4720=ORIENTED_EDGE ( 'NONE', *, *, #1773, .T. ) ;
#4723=DIRECTION ( 'NONE',  ( -0.01292394549866739996, -0.005513023399721131770, -0.9999012842304692006 ) ) ;
#4737=EDGE_CURVE ( 'NONE', #13016, #13554, #19021, .T. ) ;
#4753=EDGE_CURVE ( 'NONE', #8542, #11891, #2898, .T. ) ;
#4754=DIRECTION ( 'NONE',  ( -0.009188991635466048358, 0.7031977391749438810, -0.7109349492407661675 ) ) ;
#4757=CARTESIAN_POINT ( 'NONE',  ( -20.57109388430227881, 136.7551719540686008, -44.05520973278501629 ) ) ;
#4758=AXIS2_PLACEMENT_3D ( 'NONE', #12395, #4090, #19700 ) ;
#4772=EDGE_CURVE ( 'NONE', #12735, #14385, #5444, .T. ) ;
#4787=AXIS2_PLACEMENT_3D ( 'NONE', #9673, #14864, #11385 ) ;
#4796=CIRCLE ( 'NONE', #7776, 7.499999999999991118 ) ;
#4797=CARTESIAN_POINT ( 'NONE',  ( -50.59241450076314095, 108.3707227317548103, -45.51087538574415703 ) ) ;
#4804=DIRECTION ( 'NONE',  ( -0.01292394549866741904, -0.005513023399721091004, -0.9999012842304693116 ) ) ;
#4819=CARTESIAN_POINT ( 'NONE',  ( 48.70718024533385915, 95.27297528470670329, -45.18526822691359257 ) ) ;
#4823=DIRECTION ( 'NONE',  ( 0.9999164797902015955, 6.965998958219364448E-18, -0.01292414190464157182 ) ) ;
#4829=CARTESIAN_POINT ( 'NONE',  ( 64.42123688909094881, 144.7550503794368524, -45.19786229828635271 ) ) ;
#4832=AXIS2_PLACEMENT_3D ( 'NONE', #10395, #10509, #12356 ) ;
#4834=CARTESIAN_POINT ( 'NONE',  ( 51.12138307655921921, 113.4816418249608319, -44.85353068836323587 ) ) ;
#4838=EDGE_LOOP ( 'NONE', ( #6412, #8577, #19529, #18955 ) ) ;
#4858=CARTESIAN_POINT ( 'NONE',  ( -20.14020152772452477, -0.1201756712316815051, -10.71788091538852861 ) ) ;
#4860=EDGE_CURVE ( 'NONE', #1365, #13728, #8249, .T. ) ;
#4861=DIRECTION ( 'NONE',  ( -0.003413786507415475339, 0.9644842718275420390, -0.2641182225045781706 ) ) ;
#4869=AXIS2_PLACEMENT_3D ( 'NONE', #10637, #14107, #21088 ) ;
#4871=CIRCLE ( 'NONE', #1576, 8.000000000000005329 ) ;
#4872=EDGE_CURVE ( 'NONE', #8679, #13676, #15384, .T. ) ;
#4873=FACE_OUTER_BOUND ( 'NONE', #15891, .T. ) ;
#4876=VERTEX_POINT ( 'NONE', #22114 ) ;
#4877=ORIENTED_EDGE ( 'NONE', *, *, #19305, .F. ) ;
#4878=CARTESIAN_POINT ( 'NONE',  ( -37.14184569576254091, 95.72081062788153361, 84.97917966163161907 ) ) ;
#4891=CARTESIAN_POINT ( 'NONE',  ( 41.42451162475439475, 125.7553391191873544, -44.79586833841344173 ) ) ;
#4892=ORIENTED_EDGE ( 'NONE', *, *, #4772, .F. ) ;
#4902=CARTESIAN_POINT ( 'NONE',  ( 64.42446510409216387, 113.4816418249608034, -45.02547596916208050 ) ) ;
#4906=AXIS2_PLACEMENT_3D ( 'NONE', #16107, #8839, #2971 ) ;
#4910=CARTESIAN_POINT ( 'NONE',  ( 44.31808358225305966, 164.8106407359766763, -53.04939224934937414 ) ) ;
#4917=VECTOR ( 'NONE', #17641, 1000.000000000000000 ) ;
#4922=DIRECTION ( 'NONE',  ( -0.9999164797902015955, -6.965998958219364448E-18, 0.01292414190464157182 ) ) ;
#4928=CARTESIAN_POINT ( 'NONE',  ( 49.46305616158914376, 112.8312625773126712, -44.82851053580059641 ) ) ;
#4936=CARTESIAN_POINT ( 'NONE',  ( 49.18241401050376993, 95.63349031005608936, -45.79074433281897427 ) ) ;
#4941=AXIS2_PLACEMENT_3D ( 'NONE', #346, #238, #5498 ) ;
#4946=CARTESIAN_POINT ( 'NONE',  ( -45.96219963993937796, 168.0879242961143518, -74.15276576609245751 ) ) ;
#4960=ORIENTED_EDGE ( 'NONE', *, *, #12149, .F. ) ;
#4961=AXIS2_PLACEMENT_3D ( 'NONE', #2964, #14838, #21788 ) ;
#4968=DIRECTION ( 'NONE',  ( -7.125109674161246868E-05, 0.9999848031710253382, -0.005512562950850155054 ) ) ;
#4978=DIRECTION ( 'NONE',  ( 0.01292394549866740169, 0.005513023399719847208, 0.9999012842304693116 ) ) ;
#4981=FACE_OUTER_BOUND ( 'NONE', #2499, .T. ) ;
#4982=CARTESIAN_POINT ( 'NONE',  ( -50.96731222690930707, 189.5912335953706531, -73.54703356252615265 ) ) ;
#4985=DIRECTION ( 'NONE',  ( 7.125109674161246868E-05, -0.9999848031710252272, 0.005512562950850154186 ) ) ;
#4989=ORIENTED_EDGE ( 'NONE', *, *, #21416, .F. ) ;
#4996=EDGE_CURVE ( 'NONE', #22603, #20787, #15838, .T. ) ;
#5003=ORIENTED_EDGE ( 'NONE', *, *, #6709, .T. ) ;
#5014=CARTESIAN_POINT ( 'NONE',  ( -42.54575983488186353, 169.7656965055118974, -41.95299061980001198 ) ) ;
#5030=CARTESIAN_POINT ( 'NONE',  ( -51.39797222600954996, 113.2588685554743790, -43.52721704555492011 ) ) ;
#5032=CARTESIAN_POINT ( 'NONE',  ( 48.26683418982636908, 111.5078795592862662, -44.80575254011499453 ) ) ;
#5052=ORIENTED_EDGE ( 'NONE', *, *, #4420, .T. ) ;
#5055=CARTESIAN_POINT ( 'NONE',  ( 64.42259065992904254, 125.7553391191873544, -45.09312360222019578 ) ) ;
#5059=CARTESIAN_POINT ( 'NONE',  ( -52.93224801690938364, 189.4877715051681832, -92.28976992631349674 ) ) ;
#5069=EDGE_CURVE ( 'NONE', #2773, #6559, #2562, .T. ) ;
#5084=AXIS2_PLACEMENT_3D ( 'NONE', #13341, #4574, #11834 ) ;
#5088=FACE_OUTER_BOUND ( 'NONE', #21676, .T. ) ;
#5095=DIRECTION ( 'NONE',  ( -7.125109674161230605E-05, 0.9999848031710253382, -0.005512562950850140309 ) ) ;
#5117=VECTOR ( 'NONE', #19830, 1000.000000000000000 ) ;
#5122=EDGE_CURVE ( 'NONE', #2491, #20773, #21751, .T. ) ;
#5125=CYLINDRICAL_SURFACE ( 'NONE', #20542, 2.000000000000001332 ) ;
#5138=CARTESIAN_POINT ( 'NONE',  ( -50.59335657864021840, 108.5738102592509335, -45.58376217401134056 ) ) ;
#5146=DIRECTION ( 'NONE',  ( 0.009188991635466048358, -0.7031977391749438810, 0.7109349492407661675 ) ) ;
#5148=FACE_OUTER_BOUND ( 'NONE', #5647, .T. ) ;
#5175=PLANE ( 'NONE',  #18835 ) ;
#5179=CARTESIAN_POINT ( 'NONE',  ( -65.56436017564475094, 94.99786382055523859, -43.24343005912400173 ) ) ;
#5200=VECTOR ( 'NONE', #3538, 999.9999999999998863 ) ;
#5205=EDGE_CURVE ( 'NONE', #13022, #16435, #6589, .T. ) ;
#5207=LINE ( 'NONE', #10737, #1267 ) ;
#5212=CARTESIAN_POINT ( 'NONE',  ( -52.39628412465351914, 189.6008764489689611, -71.77933984920133526 ) ) ;
#5216=ORIENTED_EDGE ( 'NONE', *, *, #10833, .T. ) ;
#5221=FACE_OUTER_BOUND ( 'NONE', #10958, .T. ) ;
#5222=CIRCLE ( 'NONE', #4496, 4.199999999999997513 ) ;
#5235=AXIS2_PLACEMENT_3D ( 'NONE', #16975, #18890, #4644 ) ;
#5246=LINE ( 'NONE', #20994, #21592 ) ;
#5253=DIRECTION ( 'NONE',  ( -0.9999164797902015955, -6.965998958219364448E-18, 0.01292414190464157182 ) ) ;
#5263=CARTESIAN_POINT ( 'NONE',  ( 47.86827886238202723, 110.7146866689297582, -44.79622780157797735 ) ) ;
#5271=CARTESIAN_POINT ( 'NONE',  ( -48.80449223365644684, 105.5072037373731888, 92.81729778463858338 ) ) ;
#5276=EDGE_CURVE ( 'NONE', #17777, #22622, #3810, .T. ) ;
#5277=DIRECTION ( 'NONE',  ( 0.01246513159389404414, 0.2641402835564772844, 0.9644037178988117409 ) ) ;
#5286=EDGE_LOOP ( 'NONE', ( #9687, #15268, #13597, #17306 ) ) ;
#5292=DIRECTION ( 'NONE',  ( 0.9999164797902015955, 6.965998958219364448E-18, -0.01292414190464157182 ) ) ;
#5295=DIRECTION ( 'NONE',  ( -7.125109674243555432E-05, 0.9999848031710253382, -0.005512562950850175003 ) ) ;
#5297=DIRECTION ( 'NONE',  ( -7.125109674243555432E-05, 0.9999848031710253382, -0.005512562950850175003 ) ) ;
#5312=ORIENTED_EDGE ( 'NONE', *, *, #3449, .T. ) ;
#5317=CARTESIAN_POINT ( 'NONE',  ( 19.99832959580401948, 170.0000000000008242, -0.2584828380919867996 ) ) ;
#5318=CARTESIAN_POINT ( 'NONE',  ( 51.07356891511743413, 94.48610424851698042, 82.73688480180348392 ) ) ;
#5322=CARTESIAN_POINT ( 'NONE',  ( -40.91700983470048669, 95.59801226234188221, 82.80155338050317937 ) ) ;
#5337=AXIS2_PLACEMENT_3D ( 'NONE', #5980, #16121, #19863 ) ;
#5339=CARTESIAN_POINT ( 'NONE',  ( -64.07781825212431670, 106.8061942917681790, 71.76751443486088533 ) ) ;
#5341=CARTESIAN_POINT ( 'NONE',  ( -45.67464185259402853, 168.2105890667581605, -51.90496219196452188 ) ) ;
#5348=CARTESIAN_POINT ( 'NONE',  ( 51.15216422151338804, 107.4645925609455901, 69.52715930618317941 ) ) ;
#5356=CARTESIAN_POINT ( 'NONE',  ( -51.42803251223699590, 189.3893605493459233, -110.1610646708163159 ) ) ;
#5360=CARTESIAN_POINT ( 'NONE',  ( -64.99457118636311748, 170.0000000000008242, 0.8400692238025471159 ) ) ;
#5372=VERTEX_POINT ( 'NONE', #17956 ) ;
#5394=DIRECTION ( 'NONE',  ( 7.125109674161447446E-05, -0.9999848031710253382, 0.005512562950850309444 ) ) ;
#5395=ORIENTED_EDGE ( 'NONE', *, *, #881, .T. ) ;
#5398=ORIENTED_EDGE ( 'NONE', *, *, #19604, .T. ) ;
#5405=PLANE ( 'NONE',  #19093 ) ;
#5406=ORIENTED_EDGE ( 'NONE', *, *, #17818, .F. ) ;
#5407=CARTESIAN_POINT ( 'NONE',  ( -39.27191838138413260, 107.6444011096156999, 72.18501429557439053 ) ) ;
#5408=SURFACE_STYLE_FILL_AREA ( #21161 ) ;
#5412=ORIENTED_EDGE ( 'NONE', *, *, #17203, .T. ) ;
#5422=DIRECTION ( 'NONE',  ( -0.01292394549866739996, -0.005513023399721131770, -0.9999012842304692006 ) ) ;
#5424=EDGE_LOOP ( 'NONE', ( #3370, #20935, #16893, #13245, #9677, #8824, #14554, #5406, #8907, #22526, #14174, #20482, #14940, #3307, #6283 ) ) ;
#5430=CARTESIAN_POINT ( 'NONE',  ( -38.49583147354520918, 96.47889134396454835, 84.63024825845769783 ) ) ;
#5431=ADVANCED_FACE ( 'NONE', ( #11383 ), #15076, .F. ) ;
#5444=CIRCLE ( 'NONE', #5457, 95.00000000000001421 ) ;
#5452=EDGE_CURVE ( 'NONE', #10697, #2793, #9781, .T. ) ;
#5457=AXIS2_PLACEMENT_3D ( 'NONE', #920, #8016, #8141 ) ;
#5461=LINE ( 'NONE', #17681, #7007 ) ;
#5466=CARTESIAN_POINT ( 'NONE',  ( -38.81891740251079170, 107.5014370005211504, 91.63662627299856922 ) ) ;
#5474=CARTESIAN_POINT ( 'NONE',  ( -51.42803251223699590, 189.3893605493459233, -110.1610646708163159 ) ) ;
#5480=ADVANCED_FACE ( 'NONE', ( #5148 ), #4129, .T. ) ;
#5482=EDGE_CURVE ( 'NONE', #20680, #1571, #12906, .T. ) ;
#5483=CARTESIAN_POINT ( 'NONE',  ( 49.39923347825703814, 108.3707227317548529, -46.80328957620831432 ) ) ;
#5489=ORIENTED_EDGE ( 'NONE', *, *, #22256, .T. ) ;
#5497=ORIENTED_EDGE ( 'NONE', *, *, #20919, .F. ) ;
#5498=DIRECTION ( 'NONE',  ( 0.003413786507418932210, -0.9644842718275384863, 0.2641182225045910492 ) ) ;
#5507=VECTOR ( 'NONE', #4176, 1000.000000000000114 ) ;
#5512=AXIS2_PLACEMENT_3D ( 'NONE', #18565, #11672, #13514 ) ;
#5514=CARTESIAN_POINT ( 'NONE',  ( -49.00999508589215736, 110.7144623351035335, -43.54405342295051184 ) ) ;
#5520=ORIENTED_EDGE ( 'NONE', *, *, #6136, .T. ) ;
#5522=DIRECTION ( 'NONE',  ( -0.01292394549866738261, -0.005513023399719314648, -0.9999012842304692006 ) ) ;
#5527=CARTESIAN_POINT ( 'NONE',  ( -39.33507917608648086, 107.5562884034538769, 72.10905129613649933 ) ) ;
#5533=VECTOR ( 'NONE', #16393, 1000.000000000000000 ) ;
#5538=CIRCLE ( 'NONE', #15118, 2.000000000000001332 ) ;
#5539=EDGE_LOOP ( 'NONE', ( #17140, #15792 ) ) ;
#5544=CYLINDRICAL_SURFACE ( 'NONE', #2531, 2.000000000000001332 ) ;
#5549=CIRCLE ( 'NONE', #436, 8.000000000000005329 ) ;
#5560=ADVANCED_FACE ( 'NONE', ( #5717 ), #8943, .F. ) ;
#5563=ORIENTED_EDGE ( 'NONE', *, *, #16631, .T. ) ;
#5570=VECTOR ( 'NONE', #6901, 1000.000000000000000 ) ;
#5582=DIRECTION ( 'NONE',  ( -7.125109674161231961E-05, 0.9999848031710252272, -0.005512562950850142043 ) ) ;
#5586=CARTESIAN_POINT ( 'NONE',  ( -40.92874639037903961, 94.48610424851698042, 83.92603509844954601 ) ) ;
#5590=ORIENTED_EDGE ( 'NONE', *, *, #10621, .F. ) ;
#5600=VECTOR ( 'NONE', #4754, 1000.000000000000114 ) ;
#5605=CARTESIAN_POINT ( 'NONE',  ( 49.95329303650502339, 110.8261100212978363, -47.70120114633578368 ) ) ;
#5630=VECTOR ( 'NONE', #12093, 999.9999999999998863 ) ;
#5631=ORIENTED_EDGE ( 'NONE', *, *, #14699, .T. ) ;
#5636=CARTESIAN_POINT ( 'NONE',  ( -46.77031037318527495, 119.7725967263615985, 250.1981111634296155 ) ) ;
#5647=EDGE_LOOP ( 'NONE', ( #19643, #19545, #12569, #8314 ) ) ;
#5651=CARTESIAN_POINT ( 'NONE',  ( -51.17267260618272218, 110.8317321599929244, -46.39618586169468983 ) ) ;
#5652=VERTEX_POINT ( 'NONE', #20067 ) ;
#5661=AXIS2_PLACEMENT_3D ( 'NONE', #17166, #13838, #18771 ) ;
#5669=EDGE_LOOP ( 'NONE', ( #1341, #2252, #7969, #14032, #7123, #19464 ) ) ;
#5677=EDGE_CURVE ( 'NONE', #14965, #7858, #15797, .T. ) ;
#5704=CIRCLE ( 'NONE', #19998, 102.6746853779045381 ) ;
#5706=CARTESIAN_POINT ( 'NONE',  ( -46.78944003694669362, 119.3672327899910073, 248.7180851633275438 ) ) ;
#5712=CARTESIAN_POINT ( 'NONE',  ( 49.87189298987733110, 110.6628876857999302, -47.64038739181492588 ) ) ;
#5717=FACE_OUTER_BOUND ( 'NONE', #18952, .T. ) ;
#5724=DIRECTION ( 'NONE',  ( 0.01292394549866743465, 0.005513023399721021615, 0.9999012842304692006 ) ) ;
#5728=CARTESIAN_POINT ( 'NONE',  ( 41.32970315430851826, 107.3915281860326871, 70.92239337605512617 ) ) ;
#5731=ORIENTED_EDGE ( 'NONE', *, *, #62, .T. ) ;
#5732=ORIENTED_EDGE ( 'NONE', *, *, #11214, .F. ) ;
#5736=( BOUNDED_SURFACE ( )  B_SPLINE_SURFACE ( 3, 2, ( 
 ( #21176, #12241, #15690 ),
 ( #22633, #17637, #17524 ),
 ( #21068, #8753, #5322 ),
 ( #3602, #21281, #19451 ),
 ( #16156, #12581, #12359 ),
 ( #1890, #15930, #2010 ),
 ( #17767, #178, #16044 ),
 ( #5430, #280, #17879 ),
 ( #7275, #14313, #2112 ),
 ( #9104, #395, #16273 ),
 ( #9700, #16722, #5767 ),
 ( #969, #21502, #863 ),
 ( #11537, #21609, #2570 ),
 ( #2345, #741, #9578 ),
 ( #6014, #18100, #7738 ),
 ( #7955, #20243, #14989 ) ),
 .UNSPECIFIED., .F., .F., .T. ) 
 B_SPLINE_SURFACE_WITH_KNOTS ( ( 4, 2, 2, 2, 2, 2, 2, 4 ),
 ( 3, 3 ),
 ( 0.01296814958356296704, 0.01375736145185813344, 0.01454657332015329985, 0.01533578518844846625, 0.01612499705674363265, 0.01691420892503879905, 0.01770342079333396546, 0.01928184452992429826 ),
 ( 0.000000000000000000, 1.000000000000000000 ),
 .UNSPECIFIED. ) 
 GEOMETRIC_REPRESENTATION_ITEM ( )  RATIONAL_B_SPLINE_SURFACE ( (
 ( 1.000000000000000000, 0.7071067811865456854, 1.000000000000000000),
 ( 1.000000000000000000, 0.7085856290790960577, 1.000000000000000000),
 ( 1.000000000000000000, 0.7100245998945194925, 1.000000000000000000),
 ( 1.000000000000000000, 0.7128280673175965143, 1.000000000000000000),
 ( 1.000000000000000000, 0.7142069464324342087, 1.000000000000000000),
 ( 1.000000000000000000, 0.7168109644888088772, 1.000000000000000000),
 ( 1.000000000000000000, 0.7180337263083194088, 1.000000000000000000),
 ( 1.000000000000000000, 0.7203292399658924872, 1.000000000000000000),
 ( 1.000000000000000000, 0.7214053064842161911, 1.000000000000000000),
 ( 1.000000000000000000, 0.7233195371734718604, 1.000000000000000000),
 ( 1.000000000000000000, 0.7241710127918253859, 1.000000000000000000),
 ( 1.000000000000000000, 0.7256648496837366791, 1.000000000000000000),
 ( 1.000000000000000000, 0.7262924578673953802, 1.000000000000000000),
 ( 1.000000000000000000, 0.7277939499224679309, 1.000000000000000000),
 ( 1.000000000000000000, 0.7283089038925458780, 1.000000000000000000),
 ( 1.000000000000000000, 0.7282773916567022443, 1.000000000000000000) ) ) 
 REPRESENTATION_ITEM ( '' )  SURFACE ( )  );
#5738=ORIENTED_EDGE ( 'NONE', *, *, #1966, .F. ) ;
#5740=DIRECTION ( 'NONE',  ( 7.125109674161246868E-05, -0.9999848031710252272, 0.005512562950850154186 ) ) ;
#5749=CYLINDRICAL_SURFACE ( 'NONE', #4073, 7.499999999999991118 ) ;
#5767=CARTESIAN_POINT ( 'NONE',  ( -39.34031886361867691, 93.71576119831708240, 84.68445348450920562 ) ) ;
#5774=ORIENTED_EDGE ( 'NONE', *, *, #1053, .F. ) ;
#5786=CARTESIAN_POINT ( 'NONE',  ( 24.36720253925702906, 95.51270090492251086, 81.35618551405543997 ) ) ;
#5794=ORIENTED_EDGE ( 'NONE', *, *, #7471, .F. ) ;
#5797=DIRECTION ( 'NONE',  ( -0.01292394549866740343, -0.005513023399721215904, -0.9999012842304693116 ) ) ;
#5805=CIRCLE ( 'NONE', #18656, 2.000000000000001332 ) ;
#5818=VECTOR ( 'NONE', #18808, 999.9999999999998863 ) ;
#5819=DIRECTION ( 'NONE',  ( -0.01292394549866738261, -0.005513023399719314648, -0.9999012842304692006 ) ) ;
#5826=EDGE_CURVE ( 'NONE', #22315, #2844, #17839, .T. ) ;
#5828=EDGE_LOOP ( 'NONE', ( #14901, #9340, #7372, #2902 ) ) ;
#5831=VERTEX_POINT ( 'NONE', #12726 ) ;
#5833=DIRECTION ( 'NONE',  ( 0.9999164797902015955, 6.965998958219364448E-18, -0.01292414190464157182 ) ) ;
#5843=ORIENTED_EDGE ( 'NONE', *, *, #9184, .T. ) ;
#5852=ORIENTED_EDGE ( 'NONE', *, *, #14970, .T. ) ;
#5865=EDGE_LOOP ( 'NONE', ( #3735, #7563, #3487 ) ) ;
#5872=DIRECTION ( 'NONE',  ( 0.9999164797902017066, 6.965998958219364448E-18, -0.01292414190464157356 ) ) ;
#5879=EDGE_LOOP ( 'NONE', ( #18124, #7310, #20251, #20130 ) ) ;
#5888=CARTESIAN_POINT ( 'NONE',  ( -38.43592255312495354, 106.3319251612770699, 92.24984488169984331 ) ) ;
#5905=CIRCLE ( 'NONE', #21654, 3.399999999999985700 ) ;
#5906=LINE ( 'NONE', #634, #14374 ) ;
#5910=ORIENTED_EDGE ( 'NONE', *, *, #11361, .T. ) ;
#5911=CARTESIAN_POINT ( 'NONE',  ( 42.92324425022518852, 106.8061942917681790, 70.38450200964520320 ) ) ;
#5917=CARTESIAN_POINT ( 'NONE',  ( -45.96219963993937796, 168.0879242961143518, -74.15276576609245751 ) ) ;
#5932=CARTESIAN_POINT ( 'NONE',  ( 49.20623290202794919, 189.4921571640329603, -92.81436920875947294 ) ) ;
#5940=ADVANCED_FACE ( 'NONE', ( #17904 ), #7198, .F. ) ;
#5943=AXIS2_PLACEMENT_3D ( 'NONE', #14675, #13070, #16298 ) ;
#5949=CARTESIAN_POINT ( 'NONE',  ( -64.14977513578709534, 101.1708071963161615, 66.20034608127639331 ) ) ;
#5966=VERTEX_POINT ( 'NONE', #2605 ) ;
#5974=DIRECTION ( 'NONE',  ( 0.9999164797902017066, 6.965998958219365988E-18, -0.01292414190464157356 ) ) ;
#5975=CARTESIAN_POINT ( 'NONE',  ( -51.50781950266230069, 111.3281040458452082, -46.57401169717144285 ) ) ;
#5978=DIRECTION ( 'NONE',  ( 7.125109674161246868E-05, -0.9999848031710253382, 0.005512562950850155054 ) ) ;
#5979=VECTOR ( 'NONE', #764, 1000.000000000000114 ) ;
#5980=CARTESIAN_POINT ( 'NONE',  ( -51.99565694909051672, 170.0000000000000284, 0.6720553790413400508 ) ) ;
#5981=AXIS2_PLACEMENT_3D ( 'NONE', #7005, #22592, #1621 ) ;
#5983=ADVANCED_FACE ( 'NONE', ( #18568 ), #16178, .F. ) ;
#5989=CARTESIAN_POINT ( 'NONE',  ( 49.03340997568240311, 189.5897628274961164, -75.10636390159697839 ) ) ;
#5991=PLANE ( 'NONE',  #11809 ) ;
#5994=EDGE_LOOP ( 'NONE', ( #12687, #3289, #7073, #7551 ) ) ;
#5995=PLANE ( 'NONE',  #9651 ) ;
#5997=CARTESIAN_POINT ( 'NONE',  ( -51.36678610600512940, 111.1441465054529232, -46.50825084614805149 ) ) ;
#6001=AXIS2_PLACEMENT_3D ( 'NONE', #12332, #20, #19542 ) ;
#6006=ADVANCED_FACE ( 'NONE', ( #17422 ), #22434, .F. ) ;
#6010=CARTESIAN_POINT ( 'NONE',  ( 14.14224087380716455, 105.6999953372425409, 126.9762993157022777 ) ) ;
#6012=VECTOR ( 'NONE', #12777, 1000.000000000000114 ) ;
#6014=CARTESIAN_POINT ( 'NONE',  ( -37.14537067542799065, 95.89621381637979880, 85.13594009840959131 ) ) ;
#6019=TOROIDAL_SURFACE ( 'NONE', #19581, 77.00000000000002842, 2.000000000000000000 ) ;
#6033=CARTESIAN_POINT ( 'NONE',  ( 64.31463902574824942, 189.7102623349351802, -53.44513790491837568 ) ) ;
#6034=CARTESIAN_POINT ( 'NONE',  ( -23.44527677710862434, -5.346239964818074952, -10.02852836536016845 ) ) ;
#6038=CARTESIAN_POINT ( 'NONE',  ( 14.14167086503323034, 113.6998737626107641, 126.9321988120954643 ) ) ;
#6043=B_SPLINE_CURVE_WITH_KNOTS ( 'NONE', 3,
 ( #18696, #21814, #17968, #13132, #4260, #14873, #5997, #5651, #2203, #16593, #4031, #610, #21378, #11283 ),
 .UNSPECIFIED., .F., .F.,
 ( 4, 2, 2, 2, 2, 2, 4 ),
 ( 0.000000000000000000, 0.0005796598520817377968, 0.001159319704163475594, 0.001738979556245213174, 0.002318639408326951187, 0.003477959112490424613, 0.004637278816653898905 ),
 .UNSPECIFIED. ) ;
#6050=CARTESIAN_POINT ( 'NONE',  ( -19.99832959580404790, 170.0000000000008242, 0.2584828380936761705 ) ) ;
#6052=ADVANCED_FACE ( 'NONE', ( #4873 ), #8433, .F. ) ;
#6061=LINE ( 'NONE', #2397, #20514 ) ;
#6062=CIRCLE ( 'NONE', #7897, 110.5324305509042233 ) ;
#6064=DIRECTION ( 'NONE',  ( 0.01292394549866743812, 0.005513023399720639109, 0.9999012842304693116 ) ) ;
#6074=VECTOR ( 'NONE', #1642, 1000.000000000000000 ) ;
#6075=CARTESIAN_POINT ( 'NONE',  ( -42.28414214406363669, 95.00650440594678514, -43.52932268794753412 ) ) ;
#6085=VERTEX_POINT ( 'NONE', #8655 ) ;
#6087=CARTESIAN_POINT ( 'NONE',  ( -51.98136777917161311, 109.9521095004071753, -43.50144448901883720 ) ) ;
#6097=ORIENTED_EDGE ( 'NONE', *, *, #21966, .F. ) ;
#6126=CARTESIAN_POINT ( 'NONE',  ( -48.94038278341281512, 95.51270090492249665, 82.30370228625183415 ) ) ;
#6136=EDGE_CURVE ( 'NONE', #17033, #4427, #14208, .T. ) ;
#6139=ORIENTED_EDGE ( 'NONE', *, *, #12847, .F. ) ;
#6170=VECTOR ( 'NONE', #8237, 1000.000000000000000 ) ;
#6176=DIRECTION ( 'NONE',  ( 7.125109674161246868E-05, -0.9999848031710252272, 0.005512562950850154186 ) ) ;
#6200=CARTESIAN_POINT ( 'NONE',  ( -51.49911578223353814, 109.7083498255462075, -43.50633371739562705 ) ) ;
#6202=DIRECTION ( 'NONE',  ( -0.01292394549866739996, -0.005513023399721131770, -0.9999012842304692006 ) ) ;
#6205=FACE_OUTER_BOUND ( 'NONE', #19394, .T. ) ;
#6207=CARTESIAN_POINT ( 'NONE',  ( 64.31563894222803413, 189.7102623349352086, -53.44515082906027459 ) ) ;
#6208=ORIENTED_EDGE ( 'NONE', *, *, #16740, .T. ) ;
#6210=EDGE_LOOP ( 'NONE', ( #14831, #4562, #16614, #2850 ) ) ;
#6218=CARTESIAN_POINT ( 'NONE',  ( -64.99457118636313169, 170.0000000000000284, 0.8400692238016805868 ) ) ;
#6220=VECTOR ( 'NONE', #18928, 999.9999999999998863 ) ;
#6227=CARTESIAN_POINT ( 'NONE',  ( -36.79710281205949940, 121.2962013336460956, 248.0606072992719930 ) ) ;
#6230=ORIENTED_EDGE ( 'NONE', *, *, #8774, .F. ) ;
#6235=ORIENTED_EDGE ( 'NONE', *, *, #16847, .F. ) ;
#6236=LINE ( 'NONE', #13261, #9636 ) ;
#6245=EDGE_CURVE ( 'NONE', #13213, #15391, #6246, .T. ) ;
#6246=LINE ( 'NONE', #20250, #11018 ) ;
#6257=CARTESIAN_POINT ( 'NONE',  ( 47.76156380321228312, 110.4315385716095079, -44.79328732961231907 ) ) ;
#6258=CARTESIAN_POINT ( 'NONE',  ( 41.91771097984041461, 107.0053247559779805, 70.57445437474680716 ) ) ;
#6264=DIRECTION ( 'NONE',  ( 0.01292394549866738261, 0.005513023399722618428, 0.9999012842304692006 ) ) ;
#6271=CIRCLE ( 'NONE', #2599, 110.5324305509042233 ) ;
#6275=CARTESIAN_POINT ( 'NONE',  ( 64.05894960112136971, 189.6011917897851333, -73.22734637019877368 ) ) ;
#6283=ORIENTED_EDGE ( 'NONE', *, *, #19767, .T. ) ;
#6292=AXIS2_PLACEMENT_3D ( 'NONE', #3102, #12069, #1395 ) ;
#6293=DIRECTION ( 'NONE',  ( 0.01096700916508646859, -0.5290868411612599242, 0.8484968115555724388 ) ) ;
#6300=ORIENTED_EDGE ( 'NONE', *, *, #12705, .F. ) ;
#6304=ORIENTED_EDGE ( 'NONE', *, *, #292, .T. ) ;
#6307=CARTESIAN_POINT ( 'NONE',  ( -38.81316173502003863, 96.91662645125910558, 84.24247758608711933 ) ) ;
#6309=ORIENTED_EDGE ( 'NONE', *, *, #15264, .T. ) ;
#6311=DIRECTION ( 'NONE',  ( -0.01292394549866737220, -0.005513023399721000799, -0.9999012842304692006 ) ) ;
#6312=VECTOR ( 'NONE', #20691, 999.9999999999998863 ) ;
#6323=EDGE_CURVE ( 'NONE', #21650, #5831, #4056, .T. ) ;
#6327=CARTESIAN_POINT ( 'NONE',  ( -52.81114432656352875, 109.8083481694280721, -43.48992680558292534 ) ) ;
#6330=AXIS2_PLACEMENT_3D ( 'NONE', #6010, #20007, #4271 ) ;
#6333=DIRECTION ( 'NONE',  ( 0.9999164797902017066, 0.000000000000000000, -0.01292414190464157529 ) ) ;
#6340=CARTESIAN_POINT ( 'NONE',  ( -65.67450334697799974, 189.7102623349352086, -51.76499945731497121 ) ) ;
#6346=ADVANCED_FACE ( 'NONE', ( #14899 ), #19798, .T. ) ;
#6360=VERTEX_POINT ( 'NONE', #21840 ) ;
#6366=DIRECTION ( 'NONE',  ( -0.01292394549866736873, -0.005513023399717647578, -0.9999012842304690896 ) ) ;
#6373=ORIENTED_EDGE ( 'NONE', *, *, #14305, .T. ) ;
#6375=VECTOR ( 'NONE', #14801, 1000.000000000000000 ) ;
#6394=CARTESIAN_POINT ( 'NONE',  ( 41.33663990117435816, 95.22970684149694875, 83.53052428595084677 ) ) ;
#6395=FACE_OUTER_BOUND ( 'NONE', #5424, .T. ) ;
#6406=CIRCLE ( 'NONE', #533, 75.00000000000002842 ) ;
#6408=B_SPLINE_CURVE_WITH_KNOTS ( 'NONE', 3,
 ( #14265, #16348, #2525, #587, #7580, #17940, #21467, #18169, #9409, #12874, #5728, #2420, #12761, #13005, #4236, #470 ),
 .UNSPECIFIED., .F., .F.,
 ( 4, 2, 2, 2, 2, 2, 2, 4 ),
 ( -2.211772431870429045E-17, 0.0003967982407998327829, 0.0007935964815996876835, 0.001190394722399542530, 0.001587192963199397485, 0.001983991203999252440, 0.002380789444799107177, 0.003174385926398843108 ),
 .UNSPECIFIED. ) ;
#6412=ORIENTED_EDGE ( 'NONE', *, *, #4860, .F. ) ;
#6414=DIRECTION ( 'NONE',  ( -0.01292394549866739996, -0.005513023399721131770, -0.9999012842304692006 ) ) ;
#6424=ORIENTED_EDGE ( 'NONE', *, *, #17203, .F. ) ;
#6431=ADVANCED_FACE ( 'NONE', ( #22617 ), #15787, .F. ) ;
#6432=STYLED_ITEM ( 'NONE', ( #19993 ), #9632 ) ;
#6443=FACE_OUTER_BOUND ( 'NONE', #14951, .T. ) ;
#6447=DIRECTION ( 'NONE',  ( -0.9999164797902015955, -6.965998958219364448E-18, 0.01292414190464157182 ) ) ;
#6451=DIRECTION ( 'NONE',  ( -7.125109674161246868E-05, 0.9999848031710252272, -0.005512562950850154186 ) ) ;
#6457=ADVANCED_FACE ( 'NONE', ( #15910 ), #5405, .F. ) ;
#6467=ORIENTED_EDGE ( 'NONE', *, *, #21009, .F. ) ;
#6485=DIRECTION ( 'NONE',  ( -7.125109674243555432E-05, 0.9999848031710253382, -0.005512562950850175003 ) ) ;
#6490=LINE ( 'NONE', #13504, #11924 ) ;
#6494=CARTESIAN_POINT ( 'NONE',  ( -49.57489512272184129, 107.2650309926512193, 71.07430715179511083 ) ) ;
#6501=CARTESIAN_POINT ( 'NONE',  ( 42.82096601309913808, 94.49577377718297555, 82.85231139482363005 ) ) ;
#6503=CARTESIAN_POINT ( 'NONE',  ( -51.34037389809783036, 189.5966443421384611, -72.56069641891028255 ) ) ;
#6507=ORIENTED_EDGE ( 'NONE', *, *, #10083, .T. ) ;
#6512=ORIENTED_EDGE ( 'NONE', *, *, #19767, .F. ) ;
#6513=FACE_OUTER_BOUND ( 'NONE', #15526, .T. ) ;
#6519=VERTEX_POINT ( 'NONE', #1990 ) ;
#6525=FACE_OUTER_BOUND ( 'NONE', #12109, .T. ) ;
#6533=CARTESIAN_POINT ( 'NONE',  ( 51.39870305934242367, 113.4706157781613598, -46.85725176872078634 ) ) ;
#6540=DIRECTION ( 'NONE',  ( -0.01292394549866736873, -0.005513023399721228915, -0.9999012842304690896 ) ) ;
#6547=CARTESIAN_POINT ( 'NONE',  ( 51.15696624816380478, 110.0038319760128189, -44.83481546877135315 ) ) ;
#6548=VERTEX_POINT ( 'NONE', #1867 ) ;
#6553=EDGE_CURVE ( 'NONE', #18095, #18970, #14180, .T. ) ;
#6559=VERTEX_POINT ( 'NONE', #18080 ) ;
#6583=DIRECTION ( 'NONE',  ( 0.01292394549866747802, 0.005513023399721269681, 0.9999012842304692006 ) ) ;
#6585=ADVANCED_FACE ( 'NONE', ( #6525 ), #10939, .F. ) ;
#6586=DIRECTION ( 'NONE',  ( -0.01292394549866738608, -0.005513023399721785761, -0.9999012842304693116 ) ) ;
#6589=CIRCLE ( 'NONE', #19416, 3.399999999999985700 ) ;
#6590=ORIENTED_EDGE ( 'NONE', *, *, #8759, .F. ) ;
#6592=DIRECTION ( 'NONE',  ( -0.9999164797902015955, -6.965998958219364448E-18, 0.01292414190464157182 ) ) ;
#6598=FACE_OUTER_BOUND ( 'NONE', #2839, .T. ) ;
#6600=CARTESIAN_POINT ( 'NONE',  ( 44.03028354117878251, 168.0879242961143518, -75.31593853751020617 ) ) ;
#6605=CARTESIAN_POINT ( 'NONE',  ( -39.06508167816152621, 108.1171923551751917, 72.59136061629835979 ) ) ;
#6619=AXIS2_PLACEMENT_3D ( 'NONE', #6973, #22341, #6641 ) ;
#6633=CARTESIAN_POINT ( 'NONE',  ( -64.99457118636311748, 170.0000000000008242, 0.8400692238025471159 ) ) ;
#6641=DIRECTION ( 'NONE',  ( 0.01292394549866695240, 0.005513023399718316314, 0.9999012842304693116 ) ) ;
#6647=ORIENTED_EDGE ( 'NONE', *, *, #5452, .T. ) ;
#6653=DIRECTION ( 'NONE',  ( 0.9999164797902015955, 6.965998958219364448E-18, -0.01292414190464157182 ) ) ;
#6659=CARTESIAN_POINT ( 'NONE',  ( 50.20590380062862579, 109.5893650058224864, -44.82023758435901328 ) ) ;
#6662=PLANE ( 'NONE',  #15473 ) ;
#6663=LINE ( 'NONE', #2988, #14486 ) ;
#6664=DIRECTION ( 'NONE',  ( -0.01292394549866695240, -0.005513023399718316314, -0.9999012842304693116 ) ) ;
#6666=CARTESIAN_POINT ( 'NONE',  ( -50.93144557475185508, 189.6011917897851333, -71.74107005116499636 ) ) ;
#6670=ORIENTED_EDGE ( 'NONE', *, *, #13488, .F. ) ;
#6685=VECTOR ( 'NONE', #13678, 1000.000000000000000 ) ;
#6688=AXIS2_PLACEMENT_3D ( 'NONE', #19610, #19945, #7561 ) ;
#6690=CARTESIAN_POINT ( 'NONE',  ( -51.18712128330030708, 189.4975170488156380, -90.54447405611476540 ) ) ;
#6693=ORIENTED_EDGE ( 'NONE', *, *, #20555, .T. ) ;
#6697=DIRECTION ( 'NONE',  ( -7.125109674161246868E-05, 0.9999848031710253382, -0.005512562950850155054 ) ) ;
#6707=AXIS2_PLACEMENT_3D ( 'NONE', #7901, #18474, #13429 ) ;
#6709=EDGE_CURVE ( 'NONE', #2480, #7828, #8818, .T. ) ;
#6720=DIRECTION ( 'NONE',  ( -0.01246513159389404414, -0.2641402835564772289, -0.9644037178988116299 ) ) ;
#6729=ORIENTED_EDGE ( 'NONE', *, *, #20409, .T. ) ;
#6769=CARTESIAN_POINT ( 'NONE',  ( 64.38126239552605057, 111.9218655255082382, -48.29061345977370934 ) ) ;
#6776=DIRECTION ( 'NONE',  ( 0.9999164797902017066, 6.965998958219367529E-18, -0.01292414190464157182 ) ) ;
#6777=DIRECTION ( 'NONE',  ( -7.125109674161257710E-05, 0.9999848031710252272, -0.005512562950850163727 ) ) ;
#6780=CYLINDRICAL_SURFACE ( 'NONE', #12785, 1.999999999999997780 ) ;
#6789=ORIENTED_EDGE ( 'NONE', *, *, #9747, .T. ) ;
#6792=DIRECTION ( 'NONE',  ( -0.9999164797902015955, -6.965998958219364448E-18, 0.01292414190464157182 ) ) ;
#6799=ORIENTED_EDGE ( 'NONE', *, *, #10085, .T. ) ;
#6801=DIRECTION ( 'NONE',  ( -0.9999164797902017066, 0.000000000000000000, 0.01292414190463832269 ) ) ;
#6808=FACE_OUTER_BOUND ( 'NONE', #16337, .T. ) ;
#6811=EDGE_LOOP ( 'NONE', ( #6512, #6845, #20504, #9867, #18369 ) ) ;
#6813=EDGE_LOOP ( 'NONE', ( #10696, #3347, #4989 ) ) ;
#6826=CYLINDRICAL_SURFACE ( 'NONE', #1968, 1.999999999999997780 ) ;
#6828=CARTESIAN_POINT ( 'NONE',  ( -50.95823800333778308, 189.5897628274961164, -73.81394971113282111 ) ) ;
#6845=ORIENTED_EDGE ( 'NONE', *, *, #21257, .T. ) ;
#6847=EDGE_LOOP ( 'NONE', ( #9285, #17656 ) ) ;
#6848=LINE ( 'NONE', #13869, #13008 ) ;
#6851=DIRECTION ( 'NONE',  ( 0.9999164797902015955, 6.965998958219364448E-18, -0.01292414190464157182 ) ) ;
#6853=DIRECTION ( 'NONE',  ( 0.9999164797902015955, 6.965998958219364448E-18, -0.01292414190464157182 ) ) ;
#6861=AXIS2_PLACEMENT_3D ( 'NONE', #8304, #20584, #16943 ) ;
#6870=DIRECTION ( 'NONE',  ( -7.125109674243555432E-05, 0.9999848031710253382, -0.005512562950850175003 ) ) ;
#6876=CARTESIAN_POINT ( 'NONE',  ( 47.42524840967396216, 108.3817487785543108, -44.77763872393808953 ) ) ;
#6877=ORIENTED_EDGE ( 'NONE', *, *, #16268, .T. ) ;
#6897=CIRCLE ( 'NONE', #19725, 1.999999999999998446 ) ;
#6898=ORIENTED_EDGE ( 'NONE', *, *, #16589, .F. ) ;
#6901=DIRECTION ( 'NONE',  ( 0.9999164797902015955, 6.965998958219364448E-18, -0.01292414190464157182 ) ) ;
#6923=EDGE_LOOP ( 'NONE', ( #11376, #9479, #8256, #19866 ) ) ;
#6924=CARTESIAN_POINT ( 'NONE',  ( 18.69536052806380511, 189.4444907833431273, -101.0667417618365107 ) ) ;
#6936=VERTEX_POINT ( 'NONE', #12394 ) ;
#6943=LINE ( 'NONE', #22323, #6170 ) ;
#6948=B_SPLINE_CURVE_WITH_KNOTS ( 'NONE', 3,
 ( #9736, #14807, #9484, #7884, #997, #9832, #13183, #2484, #14923, #20275, #21754, #7984, #18666, #20045 ),
 .UNSPECIFIED., .F., .F.,
 ( 4, 2, 2, 2, 2, 2, 4 ),
 ( 0.000000000000000000, 0.0003932600017084012011, 0.0007865200034168024022, 0.001179780005125203712, 0.001573040006833604804, 0.002359560010250444286, 0.003146080013667283768 ),
 .UNSPECIFIED. ) ;
#6961=CARTESIAN_POINT ( 'NONE',  ( 14.14167086503323034, 113.6998737626107641, 126.9321988120954643 ) ) ;
#6964=ORIENTED_EDGE ( 'NONE', *, *, #8099, .F. ) ;
#6973=CARTESIAN_POINT ( 'NONE',  ( -50.59277787925817194, 113.4706157781613598, -45.53898929444733312 ) ) ;
#6979=CARTESIAN_POINT ( 'NONE',  ( -65.56790548363530036, 144.7550503794368524, -43.51772385068294113 ) ) ;
#6993=CARTESIAN_POINT ( 'NONE',  ( -49.75352177949782373, 112.0038634918761602, -43.54155237634173403 ) ) ;
#6997=CARTESIAN_POINT ( 'NONE',  ( 49.42508136925437867, 108.3817487785542966, -44.80348700774737836 ) ) ;
#6998=ORIENTED_EDGE ( 'NONE', *, *, #10083, .F. ) ;
#6999=CARTESIAN_POINT ( 'NONE',  ( -66.42677970909001317, 189.3893605493459233, -109.9672025422466959 ) ) ;
#7000=CIRCLE ( 'NONE', #7351, 4.199999999999997513 ) ;
#7005=CARTESIAN_POINT ( 'NONE',  ( 44.31784132852413194, 168.2105890667581605, -53.06813496338226344 ) ) ;
#7007=VECTOR ( 'NONE', #19484, 1000.000000000000114 ) ;
#7012=ORIENTED_EDGE ( 'NONE', *, *, #1069, .T. ) ;
#7031=LINE ( 'NONE', #5179, #17778 ) ;
#7035=CIRCLE ( 'NONE', #18756, 93.00000000000001421 ) ;
#7056=VERTEX_POINT ( 'NONE', #2610 ) ;
#7069=CIRCLE ( 'NONE', #12226, 77.00000000000002842 ) ;
#7073=ORIENTED_EDGE ( 'NONE', *, *, #13722, .F. ) ;
#7077=LINE ( 'NONE', #17789, #3209 ) ;
#7081=ORIENTED_EDGE ( 'NONE', *, *, #17287, .T. ) ;
#7090=DIRECTION ( 'NONE',  ( 7.125109674161238737E-05, -0.9999848031710253382, 0.005512562950850163727 ) ) ;
#7097=EDGE_CURVE ( 'NONE', #17948, #13286, #16417, .T. ) ;
#7113=AXIS2_PLACEMENT_3D ( 'NONE', #15512, #15737, #1710 ) ;
#7117=CARTESIAN_POINT ( 'NONE',  ( -50.13499642684819690, 95.43998192129494385, -44.18671329044839524 ) ) ;
#7119=DIRECTION ( 'NONE',  ( -0.01292394549866695240, -0.005513023399711377420, -0.9999012842304693116 ) ) ;
#7123=ORIENTED_EDGE ( 'NONE', *, *, #12912, .T. ) ;
#7126=CIRCLE ( 'NONE', #8954, 2.000000000000001332 ) ;
#7138=DIRECTION ( 'NONE',  ( 0.01292394549866713108, 0.005513023399725330669, 0.9999012842304692006 ) ) ;
#7139=CARTESIAN_POINT ( 'NONE',  ( 63.54062731776301121, 169.3797848675314128, -113.3289636997295275 ) ) ;
#7144=ORIENTED_EDGE ( 'NONE', *, *, #12066, .T. ) ;
#7145=EDGE_CURVE ( 'NONE', #850, #22554, #11069, .T. ) ;
#7154=CARTESIAN_POINT ( 'NONE',  ( -50.95823800333778308, 189.5897628274961164, -73.81394971113282111 ) ) ;
#7157=ORIENTED_EDGE ( 'NONE', *, *, #14013, .T. ) ;
#7161=ORIENTED_EDGE ( 'NONE', *, *, #7415, .F. ) ;
#7166=ORIENTED_EDGE ( 'NONE', *, *, #3741, .F. ) ;
#7180=DIRECTION ( 'NONE',  ( -7.125109674243555432E-05, 0.9999848031710253382, -0.005512562950850175003 ) ) ;
#7186=EDGE_CURVE ( 'NONE', #6548, #16712, #16936, .T. ) ;
#7198=PLANE ( 'NONE',  #21614 ) ;
#7218=CARTESIAN_POINT ( 'NONE',  ( -53.19734013806819206, 189.4876967392748384, -92.29990616481009624 ) ) ;
#7219=LINE ( 'NONE', #3655, #8181 ) ;
#7222=CARTESIAN_POINT ( 'NONE',  ( -48.73626655442960498, 109.8645326797279864, -43.54290528015454953 ) ) ;
#7226=VERTEX_POINT ( 'NONE', #14887 ) ;
#7230=ORIENTED_EDGE ( 'NONE', *, *, #9485, .T. ) ;
#7238=EDGE_CURVE ( 'NONE', #15636, #22552, #14420, .T. ) ;
#7244=CIRCLE ( 'NONE', #18264, 2.000000000000001332 ) ;
#7252=DIRECTION ( 'NONE',  ( -7.125109674158749138E-05, 0.9999848031710253382, -0.005512562950850162860 ) ) ;
#7257=EDGE_CURVE ( 'NONE', #15577, #6085, #14024, .T. ) ;
#7259=CARTESIAN_POINT ( 'NONE',  ( -39.06289137140529988, 108.3156947416822362, 72.76082051835628306 ) ) ;
#7260=CARTESIAN_POINT ( 'NONE',  ( 51.99565694909048830, 170.0000000000000284, -0.6720553790413839046 ) ) ;
#7267=EDGE_CURVE ( 'NONE', #8873, #13728, #20252, .T. ) ;
#7275=CARTESIAN_POINT ( 'NONE',  ( -38.40954875669835644, 96.40145467477475449, 84.69856280946498828 ) ) ;
#7285=EDGE_LOOP ( 'NONE', ( #20641, #18717, #3595, #10265 ) ) ;
#7287=AXIS2_PLACEMENT_3D ( 'NONE', #20434, #508, #12799 ) ;
#7289=ADVANCED_FACE ( 'NONE', ( #4613 ), #21725, .F. ) ;
#7295=DIRECTION ( 'NONE',  ( 0.01292394549866739996, 0.005513023399720822122, 0.9999012842304692006 ) ) ;
#7310=ORIENTED_EDGE ( 'NONE', *, *, #649, .T. ) ;
#7312=CARTESIAN_POINT ( 'NONE',  ( 40.57355171551004958, 108.0982075334647163, 198.8652726751216733 ) ) ;
#7326=CARTESIAN_POINT ( 'NONE',  ( -49.99582398951010731, 170.0000000000000284, 0.6462070952320568828 ) ) ;
#7329=LINE ( 'NONE', #7794, #19693 ) ;
#7333=CARTESIAN_POINT ( 'NONE',  ( 19.42535155401557034, 139.7551263635816952, -44.58871309782323067 ) ) ;
#7334=CARTESIAN_POINT ( 'NONE',  ( 45.19575868936945540, 125.3640259171584290, 246.9784031832207631 ) ) ;
#7339=VERTEX_POINT ( 'NONE', #17382 ) ;
#7343=ORIENTED_EDGE ( 'NONE', *, *, #3028, .F. ) ;
#7350=LINE ( 'NONE', #21362, #16617 ) ;
#7351=AXIS2_PLACEMENT_3D ( 'NONE', #6038, #2592, #6264 ) ;
#7360=CIRCLE ( 'NONE', #1861, 7.499999999999991118 ) ;
#7361=EDGE_LOOP ( 'NONE', ( #11522, #11222, #7230, #2102, #14893, #21988 ) ) ;
#7370=CARTESIAN_POINT ( 'NONE',  ( 14.14224087380716455, 105.6999953372425409, 126.9762993157022777 ) ) ;
#7372=ORIENTED_EDGE ( 'NONE', *, *, #19041, .F. ) ;
#7379=EDGE_CURVE ( 'NONE', #2060, #14939, #10581, .T. ) ;
#7384=DIRECTION ( 'NONE',  ( 0.01292394549866695240, 0.005513023399725255208, 0.9999012842304693116 ) ) ;
#7397=ADVANCED_FACE ( 'NONE', ( #1637 ), #20912, .T. ) ;
#7401=VERTEX_POINT ( 'NONE', #4829 ) ;
#7415=EDGE_CURVE ( 'NONE', #14939, #16331, #3221, .T. ) ;
#7416=AXIS2_PLACEMENT_3D ( 'NONE', #15437, #19197, #17492 ) ;
#7420=CARTESIAN_POINT ( 'NONE',  ( 14.13996083871143306, 137.6995090387153482, 126.7998973012750810 ) ) ;
#7425=VECTOR ( 'NONE', #17171, 1000.000000000000114 ) ;
#7427=ADVANCED_FACE ( 'NONE', ( #8722 ), #9982, .F. ) ;
#7434=VERTEX_POINT ( 'NONE', #12329 ) ;
#7440=FACE_BOUND ( 'NONE', #1635, .T. ) ;
#7442=VECTOR ( 'NONE', #21878, 1000.000000000000000 ) ;
#7447=EDGE_CURVE ( 'NONE', #9718, #21686, #12087, .T. ) ;
#7453=ORIENTED_EDGE ( 'NONE', *, *, #9222, .T. ) ;
#7454=DIRECTION ( 'NONE',  ( 0.003413786507415475339, -0.9644842718275420390, 0.2641182225045781706 ) ) ;
#7455=CARTESIAN_POINT ( 'NONE',  ( -49.51659781732259802, 95.13602058458445754, -43.68511678575673329 ) ) ;
#7460=CARTESIAN_POINT ( 'NONE',  ( -51.99565694909051672, 170.0000000000000284, 0.6720553790413400508 ) ) ;
#7461=CARTESIAN_POINT ( 'NONE',  ( -40.92438434402757963, 95.47920540267311651, -42.72851707616362660 ) ) ;
#7467=ORIENTED_EDGE ( 'NONE', *, *, #15841, .T. ) ;
#7471=EDGE_CURVE ( 'NONE', #22322, #20464, #21693, .T. ) ;
#7478=PLANE ( 'NONE',  #2999 ) ;
#7482=CARTESIAN_POINT ( 'NONE',  ( -10.85624112972181621, 113.6998737626107641, 127.2553023597115214 ) ) ;
#7489=CIRCLE ( 'NONE', #8569, 4.199999999999997513 ) ;
#7495=CARTESIAN_POINT ( 'NONE',  ( -46.79626760996151802, 121.2962013336460814, 248.1898487183183875 ) ) ;
#7496=AXIS2_PLACEMENT_3D ( 'NONE', #17323, #19257, #15196 ) ;
#7524=CIRCLE ( 'NONE', #20351, 7.499999999999991118 ) ;
#7530=VERTEX_POINT ( 'NONE', #7139 ) ;
#7532=EDGE_CURVE ( 'NONE', #6360, #21645, #1913, .T. ) ;
#7535=CARTESIAN_POINT ( 'NONE',  ( 20.96603472858062034, 99.74539563421258492, 74.61103786048235520 ) ) ;
#7542=VERTEX_POINT ( 'NONE', #141 ) ;
#7551=ORIENTED_EDGE ( 'NONE', *, *, #14314, .F. ) ;
#7557=AXIS2_PLACEMENT_3D ( 'NONE', #15070, #3097, #4353 ) ;
#7561=DIRECTION ( 'NONE',  ( -0.01292394549866695240, -0.005513023399725255208, -0.9999012842304693116 ) ) ;
#7563=ORIENTED_EDGE ( 'NONE', *, *, #21170, .T. ) ;
#7566=ORIENTED_EDGE ( 'NONE', *, *, #20473, .F. ) ;
#7570=ORIENTED_EDGE ( 'NONE', *, *, #2780, .T. ) ;
#7574=CARTESIAN_POINT ( 'NONE',  ( -41.27422076403988171, 95.25460172568500639, -43.11209833513134981 ) ) ;
#7580=CARTESIAN_POINT ( 'NONE',  ( 42.26887782499613877, 106.8826913590880139, 70.46105996506696556 ) ) ;
#7583=ORIENTED_EDGE ( 'NONE', *, *, #12048, .F. ) ;
#7585=DIRECTION ( 'NONE',  ( 0.009088227368120101179, 0.7109943316365099353, 0.7031390079522383818 ) ) ;
#7598=VECTOR ( 'NONE', #20702, 1000.000000000000114 ) ;
#7602=( NAMED_UNIT ( * ) PLANE_ANGLE_UNIT ( ) SI_UNIT ( $, .RADIAN. ) );
#7612=AXIS2_PLACEMENT_3D ( 'NONE', #22432, #12010, #21884 ) ;
#7613=CARTESIAN_POINT ( 'NONE',  ( 39.53412429657601734, 95.80343351084772507, -43.21010328702048042 ) ) ;
#7625=DIRECTION ( 'NONE',  ( 0.9999164797902015955, 6.965998958219364448E-18, -0.01292414190464157182 ) ) ;
#7628=ORIENTED_EDGE ( 'NONE', *, *, #16977, .T. ) ;
#7647=EDGE_CURVE ( 'NONE', #13728, #8873, #20964, .T. ) ;
#7651=DIRECTION ( 'NONE',  ( 7.125109674161246868E-05, -0.9999848031710252272, 0.005512562950850154186 ) ) ;
#7655=ORIENTED_EDGE ( 'NONE', *, *, #15264, .F. ) ;
#7664=LINE ( 'NONE', #20061, #7442 ) ;
#7665=EDGE_CURVE ( 'NONE', #12549, #17825, #14621, .T. ) ;
#7670=EDGE_LOOP ( 'NONE', ( #16502, #3473, #3074, #9546 ) ) ;
#7671=DIRECTION ( 'NONE',  ( 0.01292394549866739996, 0.005513023399721131770, 0.9999012842304692006 ) ) ;
#7673=ORIENTED_EDGE ( 'NONE', *, *, #3759, .F. ) ;
#7695=EDGE_CURVE ( 'NONE', #3576, #719, #8159, .T. ) ;
#7699=ORIENTED_EDGE ( 'NONE', *, *, #19417, .F. ) ;
#7702=PRODUCT ( 'Movable Vise Jaw Block', 'Movable Vise Jaw Block', '', ( #13552 ) ) ;
#7709=CARTESIAN_POINT ( 'NONE',  ( 49.14156507091730930, 189.5933979181235998, -74.44835251036772661 ) ) ;
#7714=ADVANCED_FACE ( 'NONE', ( #22026 ), #7928, .F. ) ;
#7717=LINE ( 'NONE', #3921, #10458 ) ;
#7723=VECTOR ( 'NONE', #19458, 999.9999999999998863 ) ;
#7724=EDGE_LOOP ( 'NONE', ( #21643, #2918, #3898, #14974 ) ) ;
#7733=CIRCLE ( 'NONE', #16192, 3.399999999999985700 ) ;
#7734=EDGE_CURVE ( 'NONE', #8312, #15577, #19977, .T. ) ;
#7738=CARTESIAN_POINT ( 'NONE',  ( -37.38783854551962804, 93.14158652660637472, 85.23980647655857013 ) ) ;
#7747=( GEOMETRIC_REPRESENTATION_CONTEXT ( 3 ) GLOBAL_UNCERTAINTY_ASSIGNED_CONTEXT ( ( #7917 ) ) GLOBAL_UNIT_ASSIGNED_CONTEXT ( ( #7908, #8139, #11252 ) ) REPRESENTATION_CONTEXT ( 'NONE', 'WORKASPACE' ) );
#7748=ORIENTED_EDGE ( 'NONE', *, *, #10071, .F. ) ;
#7749=DIRECTION ( 'NONE',  ( -0.9999164797902017066, -6.965998958219365988E-18, 0.01292414190464157356 ) ) ;
#7755=CARTESIAN_POINT ( 'NONE',  ( -22.25632012706247664, 95.51270090492249665, 81.95880486798408526 ) ) ;
#7774=EDGE_LOOP ( 'NONE', ( #6799, #15090, #16957, #286, #187 ) ) ;
#7775=CARTESIAN_POINT ( 'NONE',  ( 48.82981265512304248, 189.4975199778058368, -91.83668375125502337 ) ) ;
#7776=AXIS2_PLACEMENT_3D ( 'NONE', #3212, #17248, #15088 ) ;
#7787=ORIENTED_EDGE ( 'NONE', *, *, #22205, .F. ) ;
#7794=CARTESIAN_POINT ( 'NONE',  ( -48.56932532720185947, 144.7550503794368524, -43.73743426306185000 ) ) ;
#7802=CARTESIAN_POINT ( 'NONE',  ( -42.56847267762256593, 125.7553391191873544, -43.71024041842355246 ) ) ;
#7807=CIRCLE ( 'NONE', #19539, 7.499999999999991118 ) ;
#7818=CARTESIAN_POINT ( 'NONE',  ( -49.75187073772171686, 112.0017951520220123, -43.54156231249048403 ) ) ;
#7822=ORIENTED_EDGE ( 'NONE', *, *, #4737, .F. ) ;
#7828=VERTEX_POINT ( 'NONE', #8034 ) ;
#7834=DIRECTION ( 'NONE',  ( 0.01292394549866743812, 0.005513023399720639109, 0.9999012842304693116 ) ) ;
#7847=ORIENTED_EDGE ( 'NONE', *, *, #292, .F. ) ;
#7855=AXIS2_PLACEMENT_3D ( 'NONE', #19317, #7252, #6801 ) ;
#7856=DIRECTION ( 'NONE',  ( -7.125109674161246868E-05, 0.9999848031710252272, -0.005512562950850154186 ) ) ;
#7858=VERTEX_POINT ( 'NONE', #8366 ) ;
#7861=DIRECTION ( 'NONE',  ( 7.125109674161238737E-05, -0.9999848031710253382, 0.005512562950850163727 ) ) ;
#7865=CARTESIAN_POINT ( 'NONE',  ( -46.77184957787964237, 141.3748088146942621, 250.0790257996952164 ) ) ;
#7879=DIRECTION ( 'NONE',  ( 0.9999164797902015955, 6.965998958219364448E-18, -0.01292414190464157182 ) ) ;
#7884=CARTESIAN_POINT ( 'NONE',  ( -40.56829007148257205, 106.8542505984647306, 71.50644046503228424 ) ) ;
#7889=ORIENTED_EDGE ( 'NONE', *, *, #14984, .T. ) ;
#7897=AXIS2_PLACEMENT_3D ( 'NONE', #10813, #18048, #17715 ) ;
#7901=CARTESIAN_POINT ( 'NONE',  ( -52.99080075248789967, 169.5754971982215125, -76.32034350670481615 ) ) ;
#7908=( LENGTH_UNIT ( ) NAMED_UNIT ( * ) SI_UNIT ( .MILLI., .METRE. ) );
#7909=LINE ( 'NONE', #18690, #11914 ) ;
#7915=DIRECTION ( 'NONE',  ( -0.9999164797902017066, 0.000000000000000000, 0.01292414190463832269 ) ) ;
#7916=VERTEX_POINT ( 'NONE', #6979 ) ;
#7917=UNCERTAINTY_MEASURE_WITH_UNIT (LENGTH_MEASURE( 1.000000000000000082E-05 ), #7908, 'distance_accuracy_value', 'NONE');
#7928=CYLINDRICAL_SURFACE ( 'NONE', #13329, 4.199999999999997513 ) ;
#7930=DIRECTION ( 'NONE',  ( 0.9999164797902017066, 6.965998958219365988E-18, -0.01292414190464157356 ) ) ;
#7951=EDGE_CURVE ( 'NONE', #9196, #16304, #1287, .T. ) ;
#7955=CARTESIAN_POINT ( 'NONE',  ( -36.88402614201490337, 95.89805508694958291, 85.13090641764658528 ) ) ;
#7961=CARTESIAN_POINT ( 'NONE',  ( 50.79373001771442375, 169.4872888238259634, -93.66287481247502456 ) ) ;
#7965=CYLINDRICAL_SURFACE ( 'NONE', #18376, 75.00000000000002842 ) ;
#7966=CARTESIAN_POINT ( 'NONE',  ( -37.99682623202767928, 170.0000000000000284, 0.4911173923763579863 ) ) ;
#7969=ORIENTED_EDGE ( 'NONE', *, *, #8240, .T. ) ;
#7984=CARTESIAN_POINT ( 'NONE',  ( -39.11973256296710133, 107.9236484503692850, 72.42537321791316174 ) ) ;
#7988=ORIENTED_EDGE ( 'NONE', *, *, #9485, .F. ) ;
#8000=LINE ( 'NONE', #9847, #16251 ) ;
#8003=EDGE_CURVE ( 'NONE', #8988, #1664, #11706, .T. ) ;
#8016=DIRECTION ( 'NONE',  ( -0.9999164797902015955, -6.965998958219364448E-18, 0.01292414190464157182 ) ) ;
#8034=CARTESIAN_POINT ( 'NONE',  ( -51.40218462123966248, 189.4003865961453812, -108.1612621023553658 ) ) ;
#8041=CYLINDRICAL_SURFACE ( 'NONE', #4787, 2.000000000000001332 ) ;
#8052=ORIENTED_EDGE ( 'NONE', *, *, #21203, .T. ) ;
#8060=VECTOR ( 'NONE', #20057, 1000.000000000000000 ) ;
#8061=DIRECTION ( 'NONE',  ( 0.01292394549866738261, 0.005513023399722618428, 0.9999012842304692006 ) ) ;
#8070=CIRCLE ( 'NONE', #1124, 1.999999999999997780 ) ;
#8073=DIRECTION ( 'NONE',  ( -0.9999164797902015955, -6.965998958219364448E-18, 0.01292414190464157182 ) ) ;
#8082=CIRCLE ( 'NONE', #1115, 87.00000000000001421 ) ;
#8091=CARTESIAN_POINT ( 'NONE',  ( 48.26619062019285167, 111.5068095596782314, -44.80573832231973341 ) ) ;
#8099=EDGE_CURVE ( 'NONE', #3163, #9820, #7219, .T. ) ;
#8101=CIRCLE ( 'NONE', #21631, 7.499999999999991118 ) ;
#8105=( BOUNDED_SURFACE ( )  B_SPLINE_SURFACE ( 3, 3, ( 
 ( #7535, #8813, #1713, #1601 ),
 ( #19040, #3306, #10330, #2243 ),
 ( #5786, #14455, #8590, #9363 ),
 ( #8692, #22574, #12821, #11321 ) ),
 .UNSPECIFIED., .F., .F., .T. ) 
 B_SPLINE_SURFACE_WITH_KNOTS ( ( 4, 4 ),
 ( 4, 4 ),
 ( 0.000000000000000000, 1.000000000000000000 ),
 ( 0.000000000000000000, 1.000000000000000000 ),
 .UNSPECIFIED. ) 
 GEOMETRIC_REPRESENTATION_ITEM ( )  RATIONAL_B_SPLINE_SURFACE ( (
 ( 1.000000000000000000, 0.5185431720251972854, 0.5185431720251972854, 1.000000000000000000),
 ( 0.8047378541243652705, 0.4172913195263988628, 0.4172913195263988628, 0.8047378541243652705),
 ( 0.8047378541243652705, 0.4172913195263988628, 0.4172913195263988628, 0.8047378541243652705),
 ( 1.000000000000000000, 0.5185431720251972854, 0.5185431720251972854, 1.000000000000000000) ) ) 
 REPRESENTATION_ITEM ( '' )  SURFACE ( )  );
#8108=CARTESIAN_POINT ( 'NONE',  ( 41.75993663531772171, 94.85495732055906615, 83.18988100811523623 ) ) ;
#8111=EDGE_CURVE ( 'NONE', #21136, #18552, #7069, .T. ) ;
#8130=CARTESIAN_POINT ( 'NONE',  ( -51.07890516687701421, 106.8060942374655156, 71.59941146007480484 ) ) ;
#8131=DIRECTION ( 'NONE',  ( 7.125109674161246868E-05, -0.9999848031710252272, 0.005512562950850154186 ) ) ;
#8138=LINE ( 'NONE', #20302, #21680 ) ;
#8139=( NAMED_UNIT ( * ) PLANE_ANGLE_UNIT ( ) SI_UNIT ( $, .RADIAN. ) );
#8141=DIRECTION ( 'NONE',  ( 0.01292394549866743465, 0.005513023399721021615, 0.9999012842304692006 ) ) ;
#8156=ORIENTED_EDGE ( 'NONE', *, *, #17287, .F. ) ;
#8157=CARTESIAN_POINT ( 'NONE',  ( -52.88443356760686953, 109.6548370181895962, -43.48813313179322648 ) ) ;
#8159=CIRCLE ( 'NONE', #14044, 75.00000000000002842 ) ;
#8163=CARTESIAN_POINT ( 'NONE',  ( 49.40018710923111911, 94.98683777375578074, -46.72950894661879317 ) ) ;
#8179=CARTESIAN_POINT ( 'NONE',  ( 47.57075801145018801, 94.99786382055530964, -44.70572651227904970 ) ) ;
#8181=VECTOR ( 'NONE', #10897, 1000.000000000000000 ) ;
#8183=ADVANCED_FACE ( 'NONE', ( #9510 ), #113, .F. ) ;
#8189=VERTEX_POINT ( 'NONE', #14707 ) ;
#8197=CARTESIAN_POINT ( 'NONE',  ( -51.17277943929727968, 189.4982449580671471, -90.41261591246242801 ) ) ;
#8198=ORIENTED_EDGE ( 'NONE', *, *, #11263, .T. ) ;
#8202=CIRCLE ( 'NONE', #11133, 112.5000000000000142 ) ;
#8212=EDGE_LOOP ( 'NONE', ( #20133, #5003, #1763, #16356 ) ) ;
#8216=EDGE_LOOP ( 'NONE', ( #10146, #15839, #8482, #12667, #15850, #13501, #8833, #7081 ) ) ;
#8223=DIRECTION ( 'NONE',  ( 0.9999164797902017066, 6.965998958219365988E-18, -0.01292414190464157356 ) ) ;
#8234=DIRECTION ( 'NONE',  ( 0.003413786507415475339, -0.9644842718275420390, 0.2641182225045781706 ) ) ;
#8237=DIRECTION ( 'NONE',  ( 0.9999164797902015955, 6.965998958219364448E-18, -0.01292414190464157182 ) ) ;
#8240=EDGE_CURVE ( 'NONE', #1849, #2415, #2202, .T. ) ;
#8247=EDGE_CURVE ( 'NONE', #13913, #5652, #11585, .T. ) ;
#8249=LINE ( 'NONE', #11934, #5818 ) ;
#8252=EDGE_CURVE ( 'NONE', #4037, #9196, #11131, .T. ) ;
#8256=ORIENTED_EDGE ( 'NONE', *, *, #13178, .F. ) ;
#8260=FACE_OUTER_BOUND ( 'NONE', #8669, .T. ) ;
#8264=DIRECTION ( 'NONE',  ( 0.01292394549866738261, 0.005513023399722618428, 0.9999012842304692006 ) ) ;
#8267=CARTESIAN_POINT ( 'NONE',  ( -50.64859668917933533, 109.1804550457673884, -45.80181734348686717 ) ) ;
#8268=DIRECTION ( 'NONE',  ( -7.125109674161230605E-05, 0.9999848031710253382, -0.005512562950850140309 ) ) ;
#8270=DIRECTION ( 'NONE',  ( -0.01292394549866739996, -0.005513023399721131770, -0.9999012842304692006 ) ) ;
#8281=PLANE ( 'NONE',  #22343 ) ;
#8287=FACE_OUTER_BOUND ( 'NONE', #1899, .T. ) ;
#8288=EDGE_LOOP ( 'NONE', ( #16322, #12346, #14812, #1437 ) ) ;
#8296=FACE_OUTER_BOUND ( 'NONE', #18258, .T. ) ;
#8302=FACE_OUTER_BOUND ( 'NONE', #7724, .T. ) ;
#8304=CARTESIAN_POINT ( 'NONE',  ( -35.42010074854528767, 108.0982075334647163, 199.8475074598744357 ) ) ;
#8312=VERTEX_POINT ( 'NONE', #15852 ) ;
#8314=ORIENTED_EDGE ( 'NONE', *, *, #13656, .T. ) ;
#8322=CARTESIAN_POINT ( 'NONE',  ( 41.14038128610372524, 95.59192558790229555, 83.85389257729781320 ) ) ;
#8323=FACE_OUTER_BOUND ( 'NONE', #9672, .T. ) ;
#8326=CARTESIAN_POINT ( 'NONE',  ( -40.19002855417061681, 106.9581283947334924, 71.59385384405536001 ) ) ;
#8327=VECTOR ( 'NONE', #7671, 1000.000000000000114 ) ;
#8334=DIRECTION ( 'NONE',  ( 0.9999164797902017066, 6.965998958219365988E-18, -0.01292414190464157356 ) ) ;
#8356=CARTESIAN_POINT ( 'NONE',  ( -50.59678745519813958, 169.7436444119130101, -45.84920262148475700 ) ) ;
#8366=CARTESIAN_POINT ( 'NONE',  ( -38.79736811520099593, 127.3639955235004777, 248.0530059773089420 ) ) ;
#8367=ADVANCED_FACE ( 'NONE', ( #18924 ), #3531, .T. ) ;
#8368=DIRECTION ( 'NONE',  ( 0.9999164797902015955, 6.965998958219364448E-18, -0.01292414190464157182 ) ) ;
#8369=LINE ( 'NONE', #1290, #9412 ) ;
#8370=CIRCLE ( 'NONE', #2519, 102.6746853779045381 ) ;
#8378=LINE ( 'NONE', #11852, #15715 ) ;
#8380=ORIENTED_EDGE ( 'NONE', *, *, #6709, .F. ) ;
#8381=CARTESIAN_POINT ( 'NONE',  ( -37.99682623202767928, 170.0000000000000284, 0.4911173923763579863 ) ) ;
#8391=ORIENTED_EDGE ( 'NONE', *, *, #11904, .F. ) ;
#8393=CARTESIAN_POINT ( 'NONE',  ( -47.41227093301287709, 106.1692389898096280, 200.5308336077392823 ) ) ;
#8401=ORIENTED_EDGE ( 'NONE', *, *, #22325, .F. ) ;
#8407=LINE ( 'NONE', #15563, #10695 ) ;
#8416=CARTESIAN_POINT ( 'NONE',  ( -21.30129866354425516, 189.4444907833431273, -100.5497760856508478 ) ) ;
#8418=ADVANCED_FACE ( 'NONE', ( #8923 ), #10652, .F. ) ;
#8421=VERTEX_POINT ( 'NONE', #5356 ) ;
#8427=CARTESIAN_POINT ( 'NONE',  ( 42.95143350392208248, 94.48610424851695200, 82.84186520041141932 ) ) ;
#8428=FACE_OUTER_BOUND ( 'NONE', #18522, .T. ) ;
#8433=CYLINDRICAL_SURFACE ( 'NONE', #12864, 7.499999999999991118 ) ;
#8435=CARTESIAN_POINT ( 'NONE',  ( -39.99335306980157867, 94.48610424851698042, 83.91394493266459165 ) ) ;
#8441=ADVANCED_FACE ( 'NONE', ( #19489 ), #14355, .T. ) ;
#8445=ORIENTED_EDGE ( 'NONE', *, *, #5276, .T. ) ;
#8455=ORIENTED_EDGE ( 'NONE', *, *, #13506, .T. ) ;
#8459=CARTESIAN_POINT ( 'NONE',  ( 43.19578322759555533, 127.3639955235004777, 246.9932263411283486 ) ) ;
#8467=DIRECTION ( 'NONE',  ( 0.01292394549866739996, 0.005513023399721131770, 0.9999012842304692006 ) ) ;
#8476=ORIENTED_EDGE ( 'NONE', *, *, #15855, .T. ) ;
#8477=CARTESIAN_POINT ( 'NONE',  ( -16.77414143088337184, 138.3748544051812246, 249.7078392314084567 ) ) ;
#8479=EDGE_CURVE ( 'NONE', #1318, #20578, #3287, .T. ) ;
#8482=ORIENTED_EDGE ( 'NONE', *, *, #8111, .T. ) ;
#8494=AXIS2_PLACEMENT_3D ( 'NONE', #9792, #8496, #16808 ) ;
#8495=DIRECTION ( 'NONE',  ( -0.9999164797902017066, 0.000000000000000000, 0.01292414190463832269 ) ) ;
#8496=DIRECTION ( 'NONE',  ( -0.9999164797902017066, -6.965998958219365988E-18, 0.01292414190464157356 ) ) ;
#8497=ORIENTED_EDGE ( 'NONE', *, *, #16740, .F. ) ;
#8503=EDGE_CURVE ( 'NONE', #13554, #7434, #15060, .T. ) ;
#8520=CARTESIAN_POINT ( 'NONE',  ( 49.99439896757524338, 189.9996960634205436, -0.7564583542491037926 ) ) ;
#8537=VERTEX_POINT ( 'NONE', #5466 ) ;
#8542=VERTEX_POINT ( 'NONE', #9146 ) ;
#8544=DIRECTION ( 'NONE',  ( 0.9999164797902017066, 6.965998958219365988E-18, -0.01292414190464157356 ) ) ;
#8547=CIRCLE ( 'NONE', #14071, 4.199999999999997513 ) ;
#8561=VECTOR ( 'NONE', #11642, 1000.000000000000000 ) ;
#8568=DIRECTION ( 'NONE',  ( -7.125109674161447446E-05, 0.9999848031710253382, -0.005512562950850309444 ) ) ;
#8569=AXIS2_PLACEMENT_3D ( 'NONE', #19427, #17391, #5522 ) ;
#8570=CARTESIAN_POINT ( 'NONE',  ( -51.99565694909051672, 170.0000000000000284, 0.6720553790413400508 ) ) ;
#8572=EDGE_CURVE ( 'NONE', #16738, #14056, #8070, .T. ) ;
#8575=LINE ( 'NONE', #4902, #17795 ) ;
#8577=ORIENTED_EDGE ( 'NONE', *, *, #11320, .T. ) ;
#8589=CARTESIAN_POINT ( 'NONE',  ( -46.77099456471874817, 129.3749911766419700, 250.1451765551053654 ) ) ;
#8590=CARTESIAN_POINT ( 'NONE',  ( 21.59573423564103933, 55.00725983767638638, -133.0670891953131161 ) ) ;
#8593=DIRECTION ( 'NONE',  ( 0.9999164797902017066, 6.965998958219365988E-18, -0.01292414190464157356 ) ) ;
#8594=CARTESIAN_POINT ( 'NONE',  ( -45.67488410632294915, 171.6105373975396162, -51.92370490599741117 ) ) ;
#8601=CARTESIAN_POINT ( 'NONE',  ( 47.42520555854284225, 108.9831925648675934, -44.78095427109676052 ) ) ;
#8628=CARTESIAN_POINT ( 'NONE',  ( 42.84128820176451313, 101.1708071963161615, 64.81746289747974288 ) ) ;
#8635=CIRCLE ( 'NONE', #4961, 3.999999999999999556 ) ;
#8653=CARTESIAN_POINT ( 'NONE',  ( -50.95650037043956360, 189.5905040570864912, -73.67951233157160118 ) ) ;
#8655=CARTESIAN_POINT ( 'NONE',  ( -10.75874152970787634, 105.7413430127404439, 134.7986624950468126 ) ) ;
#8659=ORIENTED_EDGE ( 'NONE', *, *, #11484, .F. ) ;
#8661=ORIENTED_EDGE ( 'NONE', *, *, #19103, .F. ) ;
#8669=EDGE_LOOP ( 'NONE', ( #18798, #21717, #16911, #7787 ) ) ;
#8672=FACE_OUTER_BOUND ( 'NONE', #17352, .T. ) ;
#8679=VERTEX_POINT ( 'NONE', #16651 ) ;
#8692=CARTESIAN_POINT ( 'NONE',  ( 29.05310264022292444, 95.51270090492251086, 81.29561921768980426 ) ) ;
#8693=CARTESIAN_POINT ( 'NONE',  ( 64.31884524158141403, 144.7109461922390778, -53.19708549627201677 ) ) ;
#8698=LINE ( 'NONE', #21120, #13089 ) ;
#8701=CARTESIAN_POINT ( 'NONE',  ( 47.50863050553487454, 109.5713193606044200, -44.78527523389898590 ) ) ;
#8703=CARTESIAN_POINT ( 'NONE',  ( -52.59261083883858134, 113.4706157781613598, -45.51314101063805140 ) ) ;
#8715=EDGE_CURVE ( 'NONE', #17033, #2396, #7360, .T. ) ;
#8722=FACE_OUTER_BOUND ( 'NONE', #8856, .T. ) ;
#8745=VECTOR ( 'NONE', #8568, 999.9999999999998863 ) ;
#8753=CARTESIAN_POINT ( 'NONE',  ( -38.93929506000819174, 95.78282953318711179, 82.58910896792900758 ) ) ;
#8759=EDGE_CURVE ( 'NONE', #665, #1664, #13523, .T. ) ;
#8762=VECTOR ( 'NONE', #11163, 1000.000000000000114 ) ;
#8764=ADVANCED_FACE ( 'NONE', ( #15485 ), #11918, .T. ) ;
#8765=DIRECTION ( 'NONE',  ( 0.01292394549866740169, 0.005513023399720822990, 0.9999012842304693116 ) ) ;
#8770=ORIENTED_EDGE ( 'NONE', *, *, #2520, .F. ) ;
#8774=EDGE_CURVE ( 'NONE', #11284, #10034, #3158, .T. ) ;
#8778=EDGE_CURVE ( 'NONE', #2070, #14285, #19058, .T. ) ;
#8782=CARTESIAN_POINT ( 'NONE',  ( -37.41993370812568998, 108.0982075334647163, 199.8733557436837032 ) ) ;
#8788=CARTESIAN_POINT ( 'NONE',  ( 52.77990858962370169, 106.8060942374655156, 70.25701329566173570 ) ) ;
#8799=DIRECTION ( 'NONE',  ( 0.01292394549866738782, 0.005513023399721118760, 0.9999012842304692006 ) ) ;
#8813=CARTESIAN_POINT ( 'NONE',  ( 19.84463980526027527, 7.270595330592044547, -12.14917202071510971 ) ) ;
#8814=CARTESIAN_POINT ( 'NONE',  ( 49.99582398951007889, 170.0000000000000284, -0.6462070952321007367 ) ) ;
#8818=CIRCLE ( 'NONE', #21649, 110.5324305509042233 ) ;
#8824=ORIENTED_EDGE ( 'NONE', *, *, #10767, .T. ) ;
#8825=CARTESIAN_POINT ( 'NONE',  ( 49.97753088104515484, 110.8699366255535637, -47.71756500317012240 ) ) ;
#8833=ORIENTED_EDGE ( 'NONE', *, *, #32, .T. ) ;
#8839=DIRECTION ( 'NONE',  ( 0.9999164797902017066, 6.965998958219365988E-18, -0.01292414190464157356 ) ) ;
#8840=ORIENTED_EDGE ( 'NONE', *, *, #13604, .F. ) ;
#8846=CONICAL_SURFACE ( 'NONE', #9591, 3.399999999999985700, 1.029744258676653201 ) ;
#8849=DIRECTION ( 'NONE',  ( 0.01292394549866739996, 0.005513023399721131770, 0.9999012842304692006 ) ) ;
#8856=EDGE_LOOP ( 'NONE', ( #11986, #20886, #11431 ) ) ;
#8857=LINE ( 'NONE', #12438, #6012 ) ;
#8873=VERTEX_POINT ( 'NONE', #185 ) ;
#8876=AXIS2_PLACEMENT_3D ( 'NONE', #20036, #20268, #990 ) ;
#8881=CARTESIAN_POINT ( 'NONE',  ( 51.05126519560737108, 95.51270090492249665, 81.01128809578769108 ) ) ;
#8895=CARTESIAN_POINT ( 'NONE',  ( 49.39923347825703814, 108.3707227317548529, -46.80328957620831432 ) ) ;
#8896=CYLINDRICAL_SURFACE ( 'NONE', #22022, 1.999999999999997780 ) ;
#8903=VECTOR ( 'NONE', #7879, 1000.000000000000000 ) ;
#8907=ORIENTED_EDGE ( 'NONE', *, *, #22325, .T. ) ;
#8913=ORIENTED_EDGE ( 'NONE', *, *, #7379, .T. ) ;
#8918=ORIENTED_EDGE ( 'NONE', *, *, #21673, .T. ) ;
#8919=EDGE_CURVE ( 'NONE', #19509, #17777, #2120, .T. ) ;
#8921=EDGE_CURVE ( 'NONE', #163, #17125, #7733, .T. ) ;
#8923=FACE_OUTER_BOUND ( 'NONE', #4219, .T. ) ;
#8933=EDGE_CURVE ( 'NONE', #15010, #9718, #3611, .T. ) ;
#8938=CARTESIAN_POINT ( 'NONE',  ( 51.18612362345588451, 111.9218655255083235, -48.12006336945275820 ) ) ;
#8943=CYLINDRICAL_SURFACE ( 'NONE', #12110, 2.009999999999996678 ) ;
#8944=ORIENTED_EDGE ( 'NONE', *, *, #20919, .T. ) ;
#8952=DIRECTION ( 'NONE',  ( 7.125109674161246868E-05, -0.9999848031710253382, 0.005512562950850155054 ) ) ;
#8954=AXIS2_PLACEMENT_3D ( 'NONE', #8703, #17236, #7119 ) ;
#8958=CIRCLE ( 'NONE', #18870, 7.921742784567028295 ) ;
#8959=DIRECTION ( 'NONE',  ( 0.01292394549866739996, 0.005513023399720822122, 0.9999012842304692006 ) ) ;
#8961=EDGE_LOOP ( 'NONE', ( #19330, #4244, #12826, #16318 ) ) ;
#8984=ORIENTED_EDGE ( 'NONE', *, *, #8479, .T. ) ;
#8988=VERTEX_POINT ( 'NONE', #8895 ) ;
#8991=VERTEX_POINT ( 'NONE', #12594 ) ;
#8993=CARTESIAN_POINT ( 'NONE',  ( 47.39680884166017449, 144.7440243326373945, -46.97795445436837980 ) ) ;
#8998=FACE_OUTER_BOUND ( 'NONE', #15035, .T. ) ;
#9000=CIRCLE ( 'NONE', #5337, 75.00000000000002842 ) ;
#9010=ORIENTED_EDGE ( 'NONE', *, *, #12797, .T. ) ;
#9014=DIRECTION ( 'NONE',  ( -7.125109674243555432E-05, 0.9999848031710253382, -0.005512562950850175003 ) ) ;
#9025=ORIENTED_EDGE ( 'NONE', *, *, #21950, .F. ) ;
#9054=ADVANCED_FACE ( 'NONE', ( #21951 ), #7965, .T. ) ;
#9062=ORIENTED_EDGE ( 'NONE', *, *, #14777, .F. ) ;
#9079=DIRECTION ( 'NONE',  ( -0.9999164797902017066, -6.965998958219367529E-18, 0.01292414190464157182 ) ) ;
#9082=CARTESIAN_POINT ( 'NONE',  ( -40.07458683857907289, 107.0042576524874818, 71.63327710005648896 ) ) ;
#9083=LINE ( 'NONE', #16371, #4570 ) ;
#9086=ORIENTED_EDGE ( 'NONE', *, *, #1139, .T. ) ;
#9096=ORIENTED_EDGE ( 'NONE', *, *, #1509, .T. ) ;
#9099=DIRECTION ( 'NONE',  ( -0.01292394549866740690, -0.005513023399721241925, -0.9999012842304693116 ) ) ;
#9101=LINE ( 'NONE', #8881, #13189 ) ;
#9103=CARTESIAN_POINT ( 'NONE',  ( -38.79722561300751238, 125.3640259171584290, 248.0640311032106524 ) ) ;
#9104=CARTESIAN_POINT ( 'NONE',  ( -38.22145853964982365, 96.26286894743961398, 84.82045450040972412 ) ) ;
#9105=CIRCLE ( 'NONE', #12058, 7.499999999999991118 ) ;
#9119=VERTEX_POINT ( 'NONE', #14665 ) ;
#9120=DIRECTION ( 'NONE',  ( 7.125109674161246868E-05, -0.9999848031710252272, 0.005512562950850154186 ) ) ;
#9128=DIRECTION ( 'NONE',  ( 0.9999164797902015955, 6.965998958219364448E-18, -0.01292414190464157182 ) ) ;
#9134=VERTEX_POINT ( 'NONE', #2465 ) ;
#9135=EDGE_LOOP ( 'NONE', ( #1005, #21061, #9355, #6235 ) ) ;
#9138=CARTESIAN_POINT ( 'NONE',  ( 50.94927467532792775, 107.7466302394140172, 69.13694936332524321 ) ) ;
#9146=CARTESIAN_POINT ( 'NONE',  ( 43.19592572978904599, 125.3640259171584290, 247.0042514670300591 ) ) ;
#9147=LINE ( 'NONE', #12396, #13575 ) ;
#9150=FACE_OUTER_BOUND ( 'NONE', #20714, .T. ) ;
#9162=DIRECTION ( 'NONE',  ( -0.01246513159389404414, -0.2641402835564772844, -0.9644037178988117409 ) ) ;
#9163=CARTESIAN_POINT ( 'NONE',  ( -50.40543294395669704, 95.70122931221760609, -44.61497156429899746 ) ) ;
#9166=LINE ( 'NONE', #7333, #22502 ) ;
#9170=VECTOR ( 'NONE', #16724, 1000.000000000000000 ) ;
#9172=PRODUCT_DEFINITION_FORMATION_WITH_SPECIFIED_SOURCE ( 'ANY', '', #7702, .NOT_KNOWN. ) ;
#9184=EDGE_CURVE ( 'NONE', #8189, #21685, #11546, .T. ) ;
#9186=FACE_OUTER_BOUND ( 'NONE', #7361, .T. ) ;
#9187=AXIS2_PLACEMENT_3D ( 'NONE', #2824, #8544, #4537 ) ;
#9192=ORIENTED_EDGE ( 'NONE', *, *, #16690, .T. ) ;
#9196=VERTEX_POINT ( 'NONE', #7865 ) ;
#9205=EDGE_CURVE ( 'NONE', #2746, #7542, #9461, .T. ) ;
#9209=EDGE_CURVE ( 'NONE', #6936, #8421, #20211, .T. ) ;
#9213=VERTEX_POINT ( 'NONE', #2913 ) ;
#9215=FACE_BOUND ( 'NONE', #20477, .T. ) ;
#9222=EDGE_CURVE ( 'NONE', #21883, #13585, #1152, .T. ) ;
#9228=LINE ( 'NONE', #11416, #11019 ) ;
#9230=VECTOR ( 'NONE', #6202, 1000.000000000000114 ) ;
#9243=VECTOR ( 'NONE', #2166, 1000.000000000000000 ) ;
#9244=CYLINDRICAL_SURFACE ( 'NONE', #2743, 110.5324305509042233 ) ;
#9248=DIRECTION ( 'NONE',  ( 0.01292394549866740169, 0.005513023399720822990, 0.9999012842304693116 ) ) ;
#9254=ORIENTED_EDGE ( 'NONE', *, *, #16389, .T. ) ;
#9261=LINE ( 'NONE', #16310, #18774 ) ;
#9285=ORIENTED_EDGE ( 'NONE', *, *, #13839, .F. ) ;
#9286=DIRECTION ( 'NONE',  ( -0.9999164797902015955, -6.965998958219364448E-18, 0.01292414190464157182 ) ) ;
#9288=CARTESIAN_POINT ( 'NONE',  ( 51.38234815825344270, 111.9218655255082524, -48.12259961501336392 ) ) ;
#9291=LINE ( 'NONE', #340, #9243 ) ;
#9295=VECTOR ( 'NONE', #11104, 999.9999999999998863 ) ;
#9298=LINE ( 'NONE', #19845, #14533 ) ;
#9312=DIRECTION ( 'NONE',  ( 7.125109674161246868E-05, -0.9999848031710252272, 0.005512562950850154186 ) ) ;
#9328=CYLINDRICAL_SURFACE ( 'NONE', #4197, 2.000000000000001332 ) ;
#9335=ORIENTED_EDGE ( 'NONE', *, *, #8933, .T. ) ;
#9340=ORIENTED_EDGE ( 'NONE', *, *, #12902, .T. ) ;
#9343=EDGE_CURVE ( 'NONE', #2512, #13022, #5461, .T. ) ;
#9354=LINE ( 'NONE', #18436, #5533 ) ;
#9355=ORIENTED_EDGE ( 'NONE', *, *, #8240, .F. ) ;
#9362=DIRECTION ( 'NONE',  ( 7.125109674161246868E-05, -0.9999848031710252272, 0.005512562950850154186 ) ) ;
#9363=CARTESIAN_POINT ( 'NONE',  ( 21.90540070143018525, 189.4003865961453528, -109.1087788745517599 ) ) ;
#9367=CARTESIAN_POINT ( 'NONE',  ( 39.99665919160806027, 170.0000000000000284, -0.5169656761856848970 ) ) ;
#9375=CARTESIAN_POINT ( 'NONE',  ( 14.08739029393882802, 113.6767190643319196, 122.7326134183275173 ) ) ;
#9385=ORIENTED_EDGE ( 'NONE', *, *, #14970, .F. ) ;
#9396=CARTESIAN_POINT ( 'NONE',  ( -49.85669660544819948, 95.27192509958106825, -43.90954682546798438 ) ) ;
#9408=ORIENTED_EDGE ( 'NONE', *, *, #7257, .F. ) ;
#9409=CARTESIAN_POINT ( 'NONE',  ( 41.59445599892145395, 107.1767044522904939, 70.73012046083394466 ) ) ;
#9412=VECTOR ( 'NONE', #6447, 1000.000000000000000 ) ;
#9420=DIRECTION ( 'NONE',  ( 0.01292394549866743812, 0.005513023399720639109, 0.9999012842304693116 ) ) ;
#9422=ORIENTED_EDGE ( 'NONE', *, *, #18226, .F. ) ;
#9425=CARTESIAN_POINT ( 'NONE',  ( 53.19494802549758106, 127.3639955235004777, 246.8639849220819542 ) ) ;
#9433=CARTESIAN_POINT ( 'NONE',  ( 39.76222920527046512, 105.5861410271771916, 91.72774381316284575 ) ) ;
#9447=CARTESIAN_POINT ( 'NONE',  ( 40.36543714644568581, 95.16167471844536863, -44.32834889262264255 ) ) ;
#9452=ORIENTED_EDGE ( 'NONE', *, *, #2553, .F. ) ;
#9453=DIRECTION ( 'NONE',  ( 0.9999164797902015955, 6.965998958219364448E-18, -0.01292414190464157182 ) ) ;
#9459=ADVANCED_FACE ( 'NONE', ( #9489 ), #18647, .F. ) ;
#9461=LINE ( 'NONE', #20254, #12144 ) ;
#9469=CIRCLE ( 'NONE', #3233, 2.000000000000001332 ) ;
#9479=ORIENTED_EDGE ( 'NONE', *, *, #19604, .F. ) ;
#9480=EDGE_CURVE ( 'NONE', #16435, #13022, #5905, .T. ) ;
#9484=CARTESIAN_POINT ( 'NONE',  ( -40.82592696026183887, 106.8159614793892018, 71.47568422908058494 ) ) ;
#9485=EDGE_CURVE ( 'NONE', #14385, #21650, #11796, .T. ) ;
#9489=FACE_OUTER_BOUND ( 'NONE', #19333, .T. ) ;
#9499=VERTEX_POINT ( 'NONE', #21642 ) ;
#9510=FACE_OUTER_BOUND ( 'NONE', #312, .T. ) ;
#9513=ORIENTED_EDGE ( 'NONE', *, *, #20409, .F. ) ;
#9518=ORIENTED_EDGE ( 'NONE', *, *, #4753, .F. ) ;
#9523=CARTESIAN_POINT ( 'NONE',  ( 49.99582398951007889, 170.0000000000000284, -0.6462070952321007367 ) ) ;
#9535=CARTESIAN_POINT ( 'NONE',  ( -51.53950506418888722, 113.3113159538933559, -43.52567687456358669 ) ) ;
#9539=ORIENTED_EDGE ( 'NONE', *, *, #16690, .F. ) ;
#9546=ORIENTED_EDGE ( 'NONE', *, *, #18894, .F. ) ;
#9554=CARTESIAN_POINT ( 'NONE',  ( -38.76986306108200608, 107.0090700318704933, 91.89681970336006600 ) ) ;
#9559=CARTESIAN_POINT ( 'NONE',  ( 41.02615909384066839, 106.6902466465767105, 92.47289523622401930 ) ) ;
#9574=VECTOR ( 'NONE', #5095, 999.9999999999998863 ) ;
#9578=CARTESIAN_POINT ( 'NONE',  ( -37.92407594442742180, 93.21315326087319875, 85.17437120064224132 ) ) ;
#9585=CARTESIAN_POINT ( 'NONE',  ( 44.03028354117878251, 168.0879242961143518, -75.31593853751020617 ) ) ;
#9591=AXIS2_PLACEMENT_3D ( 'NONE', #9585, #16619, #2698 ) ;
#9608=CARTESIAN_POINT ( 'NONE',  ( -34.77131261570284693, 119.7725967263615985, 250.0430214605738968 ) ) ;
#9625=VERTEX_POINT ( 'NONE', #10717 ) ;
#9626=CIRCLE ( 'NONE', #12868, 1.999999999999973799 ) ;
#9631=VECTOR ( 'NONE', #13708, 1000.000000000000000 ) ;
#9632=MANIFOLD_SOLID_BREP ( 'Stock-MAS-425-1', #10036 ) ;
#9636=VECTOR ( 'NONE', #4502, 999.9999999999998863 ) ;
#9638=DIRECTION ( 'NONE',  ( 0.9999164797902015955, 6.965998958219364448E-18, -0.01292414190464157182 ) ) ;
#9646=CARTESIAN_POINT ( 'NONE',  ( -41.39699765238108853, 125.7553391191873544, -43.72538199251495428 ) ) ;
#9648=ORIENTED_EDGE ( 'NONE', *, *, #11390, .T. ) ;
#9651=AXIS2_PLACEMENT_3D ( 'NONE', #14870, #3920, #21924 ) ;
#9660=VERTEX_POINT ( 'NONE', #13033 ) ;
#9663=CARTESIAN_POINT ( 'NONE',  ( -50.94859746947806656, 110.3466764521169807, -46.22168700684313336 ) ) ;
#9665=DIRECTION ( 'NONE',  ( 7.125109674161246868E-05, -0.9999848031710252272, 0.005512562950850154186 ) ) ;
#9671=CARTESIAN_POINT ( 'NONE',  ( 64.42223680557074772, 144.7550503794368524, -45.19787522242825162 ) ) ;
#9672=EDGE_LOOP ( 'NONE', ( #16771, #4065, #9518, #3285 ) ) ;
#9673=CARTESIAN_POINT ( 'NONE',  ( 41.44900574491364154, 144.7660764262362818, -42.90080446601865560 ) ) ;
#9677=ORIENTED_EDGE ( 'NONE', *, *, #3759, .T. ) ;
#9687=ORIENTED_EDGE ( 'NONE', *, *, #1053, .T. ) ;
#9693=LINE ( 'NONE', #16603, #17402 ) ;
#9700=CARTESIAN_POINT ( 'NONE',  ( -38.11897055289185232, 96.20077349746044604, 84.87487045055679857 ) ) ;
#9701=EDGE_CURVE ( 'NONE', #9820, #18018, #9083, .T. ) ;
#9709=AXIS2_PLACEMENT_3D ( 'NONE', #6961, #14467, #13985 ) ;
#9713=DIRECTION ( 'NONE',  ( 0.9999164797902015955, 6.965998958219364448E-18, -0.01292414190464157182 ) ) ;
#9718=VERTEX_POINT ( 'NONE', #21262 ) ;
#9720=EDGE_CURVE ( 'NONE', #4427, #20375, #7524, .T. ) ;
#9728=CARTESIAN_POINT ( 'NONE',  ( 49.40009966013455056, 96.21415597129798414, -46.73627471826173974 ) ) ;
#9736=CARTESIAN_POINT ( 'NONE',  ( -41.08973838174756565, 106.8061942917681790, 71.47038841247318430 ) ) ;
#9739=CARTESIAN_POINT ( 'NONE',  ( 23.22251776072470619, 138.3748544051812246, 249.1908735552227938 ) ) ;
#9747=EDGE_CURVE ( 'NONE', #22315, #13904, #7717, .T. ) ;
#9751=DIRECTION ( 'NONE',  ( 0.01292394549866743812, 0.005513023399720639109, 0.9999012842304693116 ) ) ;
#9752=DIRECTION ( 'NONE',  ( 0.01292394549866740169, 0.005513023399720822990, 0.9999012842304693116 ) ) ;
#9755=DIRECTION ( 'NONE',  ( 0.9999164797902015955, 6.965998958219364448E-18, -0.01292414190464157182 ) ) ;
#9757=CARTESIAN_POINT ( 'NONE',  ( -38.90493699201700650, 97.20305277476600736, 83.98778727448713255 ) ) ;
#9765=ADVANCED_FACE ( 'NONE', ( #10941 ), #9328, .T. ) ;
#9769=EDGE_LOOP ( 'NONE', ( #17282, #1080, #21971, #15618, #22338 ) ) ;
#9772=CARTESIAN_POINT ( 'NONE',  ( -51.34796203869380093, 109.5896734486573791, -43.50763308276343366 ) ) ;
#9774=CARTESIAN_POINT ( 'NONE',  ( 63.56236266363622889, 189.3893605493459233, -111.6473409898501075 ) ) ;
#9776=DIRECTION ( 'NONE',  ( 0.01292394549866739996, 0.005513023399720822122, 0.9999012842304692006 ) ) ;
#9779=EDGE_CURVE ( 'NONE', #3163, #11891, #12312, .T. ) ;
#9781=LINE ( 'NONE', #9883, #1835 ) ;
#9792=CARTESIAN_POINT ( 'NONE',  ( 65.83936723693913962, 101.1708071963161615, 64.52020763367299594 ) ) ;
#9802=CARTESIAN_POINT ( 'NONE',  ( -10.85624112972181621, 113.6998737626107641, 127.2553023597115214 ) ) ;
#9807=ORIENTED_EDGE ( 'NONE', *, *, #18333, .F. ) ;
#9808=CARTESIAN_POINT ( 'NONE',  ( 51.07356891511743413, 94.48610424851698042, 82.73688480180349814 ) ) ;
#9816=CARTESIAN_POINT ( 'NONE',  ( -49.99582398951009310, 170.0000000000008242, 0.6462070952329234119 ) ) ;
#9820=VERTEX_POINT ( 'NONE', #11626 ) ;
#9821=CIRCLE ( 'NONE', #18615, 8.000000000000007105 ) ;
#9822=CARTESIAN_POINT ( 'NONE',  ( 40.97857920176954849, 107.9236484503692708, 71.39008480283784763 ) ) ;
#9824=ORIENTED_EDGE ( 'NONE', *, *, #8778, .F. ) ;
#9830=CYLINDRICAL_SURFACE ( 'NONE', #5512, 2.000000000000001332 ) ;
#9832=CARTESIAN_POINT ( 'NONE',  ( -40.19568481792634884, 106.9589643049705074, 71.59466866354080139 ) ) ;
#9839=ORIENTED_EDGE ( 'NONE', *, *, #3741, .T. ) ;
#9847=CARTESIAN_POINT ( 'NONE',  ( -46.77184957787964237, 141.3748088146942621, 250.0790257996952164 ) ) ;
#9849=CARTESIAN_POINT ( 'NONE',  ( 41.22223050257357357, 121.3072273804455250, 249.0523267991708849 ) ) ;
#9850=CARTESIAN_POINT ( 'NONE',  ( -45.96219963993937796, 168.0879242961143518, -74.15276576609245751 ) ) ;
#9867=ORIENTED_EDGE ( 'NONE', *, *, #6245, .T. ) ;
#9871=CYLINDRICAL_SURFACE ( 'NONE', #15247, 4.199999999999997513 ) ;
#9877=DIRECTION ( 'NONE',  ( 0.9999164797902015955, 6.965998958219364448E-18, -0.01292414190464157182 ) ) ;
#9882=ORIENTED_EDGE ( 'NONE', *, *, #9209, .F. ) ;
#9883=CARTESIAN_POINT ( 'NONE',  ( -16.77414143088337184, 138.3748544051812246, 249.7078392314084567 ) ) ;
#9906=AXIS2_PLACEMENT_3D ( 'NONE', #2905, #3230, #20361 ) ;
#9914=AXIS2_PLACEMENT_3D ( 'NONE', #17208, #12040, #20984 ) ;
#9916=CARTESIAN_POINT ( 'NONE',  ( -51.17105351027176141, 189.4989811950858609, -90.27908403945292548 ) ) ;
#9917=DIRECTION ( 'NONE',  ( 0.9999164797902015955, 6.965998958219364448E-18, -0.01292414190464157182 ) ) ;
#9919=CARTESIAN_POINT ( 'NONE',  ( -40.89051693738994686, 95.45168806188145538, 82.94916985812750454 ) ) ;
#9923=ORIENTED_EDGE ( 'NONE', *, *, #21388, .T. ) ;
#9936=CARTESIAN_POINT ( 'NONE',  ( -49.84871199900936745, 107.0846990171262689, 71.28987068907396463 ) ) ;
#9945=CARTESIAN_POINT ( 'NONE',  ( 63.56236266363622889, 189.3893605493459233, -111.6473409898501075 ) ) ;
#9960=CARTESIAN_POINT ( 'NONE',  ( 19.99832959580401948, 170.0000000000008242, -0.2584828380919867996 ) ) ;
#9968=DIRECTION ( 'NONE',  ( 0.01292394549866738608, 0.005513023399721785761, 0.9999012842304693116 ) ) ;
#9982=CONICAL_SURFACE ( 'NONE', #11086, 3.399999999999985700, 1.029744258676653201 ) ;
#9984=LINE ( 'NONE', #21593, #3319 ) ;
#9986=DIRECTION ( 'NONE',  ( -7.125109674158749138E-05, 0.9999848031710253382, -0.005512562950850162860 ) ) ;
#9995=CARTESIAN_POINT ( 'NONE',  ( -52.56646033833638398, 109.2346207959984241, -43.48992611560825594 ) ) ;
#10011=AXIS2_PLACEMENT_3D ( 'NONE', #14756, #20099, #14972 ) ;
#10017=AXIS2_PLACEMENT_3D ( 'NONE', #9850, #9752, #16874 ) ;
#10021=EDGE_CURVE ( 'NONE', #2415, #9625, #6062, .T. ) ;
#10026=AXIS2_PLACEMENT_3D ( 'NONE', #8381, #2991, #15316 ) ;
#10034=VERTEX_POINT ( 'NONE', #10685 ) ;
#10036=CLOSED_SHELL ( 'NONE', ( #6052, #14747, #10499, #21183, #14133, #15592, #13580, #20570, #13292, #20080, #16998, #18740, #16786, #11469, #8183, #3374, #20453, #10877, #18803, #6457, #12883, #17447, #10921, #10331, #18480, #19729, #5940, #22656, #21058, #21588, #12625, #5431, #1158, #20420, #20221, #21137, #208, #7427, #3055, #17921, #14685, #6006, #8418, #9054, #22014, #18716, #10125, #10747, #14268, #14449, #4560, #22185, #15274, #999, #2486, #16717, #6431, #811, #13201, #8367, #16730, #9459, #12620, #21997, #6585, #3524, #19709, #5983, #16146, #15765, #16110, #547, #17807, #11371, #6346, #3739, #22285, #8764, #7397, #19449, #8441, #14152, #22274, #944, #9765, #22630, #22087, #10932, #2835, #11068, #12511, #14503, #2113, #5480, #2151, #21687, #978, #18775, #15825, #4598, #10487, #5560, #19890, #12606, #7289, #21333, #1817, #7714, #14589, #21288 ) ) ;
#10042=CARTESIAN_POINT ( 'NONE',  ( 64.99457118636310327, 170.0000000000000284, -0.8400692238017243296 ) ) ;
#10049=ORIENTED_EDGE ( 'NONE', *, *, #19074, .T. ) ;
#10052=LINE ( 'NONE', #1547, #175 ) ;
#10058=EDGE_CURVE ( 'NONE', #21686, #2719, #3858, .T. ) ;
#10059=CARTESIAN_POINT ( 'NONE',  ( -50.81567181550707346, 106.8152932104169537, 71.58674244103214335 ) ) ;
#10060=DIRECTION ( 'NONE',  ( -0.008899921406766564749, 0.7251151399516315710, -0.6885701309321218266 ) ) ;
#10068=FACE_OUTER_BOUND ( 'NONE', #6923, .T. ) ;
#10071=EDGE_CURVE ( 'NONE', #6559, #8991, #193, .T. ) ;
#10077=CARTESIAN_POINT ( 'NONE',  ( -39.66554348713765421, 94.53068483135839983, 83.95012769032760502 ) ) ;
#10081=DIRECTION ( 'NONE',  ( 0.9999164797902015955, 6.965998958219364448E-18, -0.01292414190464157182 ) ) ;
#10083=EDGE_CURVE ( 'NONE', #5372, #16712, #9298, .T. ) ;
#10085=EDGE_CURVE ( 'NONE', #18095, #1703, #3667, .T. ) ;
#10106=CARTESIAN_POINT ( 'NONE',  ( 49.99582398951007889, 170.0000000000000284, -0.6462070952321007367 ) ) ;
#10117=CARTESIAN_POINT ( 'NONE',  ( -48.56673365018540522, 108.3817487785542824, -43.53692110109249569 ) ) ;
#10119=CARTESIAN_POINT ( 'NONE',  ( 48.79964398845571338, 112.2287212901250228, -44.81661363440452561 ) ) ;
#10125=ADVANCED_FACE ( 'NONE', ( #21894 ), #20410, .T. ) ;
#10144=CARTESIAN_POINT ( 'NONE',  ( 49.97599159607656816, 113.1437488774104594, -44.83686325422981156 ) ) ;
#10146=ORIENTED_EDGE ( 'NONE', *, *, #10316, .F. ) ;
#10150=LINE ( 'NONE', #8520, #22116 ) ;
#10167=CARTESIAN_POINT ( 'NONE',  ( 41.86260591032142742, 94.79175134113202716, 83.13175616242061494 ) ) ;
#10176=VERTEX_POINT ( 'NONE', #18592 ) ;
#10189=CIRCLE ( 'NONE', #3572, 95.00000000000001421 ) ;
#10190=CARTESIAN_POINT ( 'NONE',  ( 39.45066905836480942, 123.7663955596447352, -42.75919236024152070 ) ) ;
#10203=EDGE_CURVE ( 'NONE', #3163, #4059, #8635, .T. ) ;
#10211=DIRECTION ( 'NONE',  ( 7.125109674161246868E-05, -0.9999848031710252272, 0.005512562950850154186 ) ) ;
#10216=LINE ( 'NONE', #8693, #6685 ) ;
#10226=CARTESIAN_POINT ( 'NONE',  ( 50.40377811878446579, 111.4597656593367958, -47.93967249470197345 ) ) ;
#10227=ORIENTED_EDGE ( 'NONE', *, *, #19041, .T. ) ;
#10232=EDGE_CURVE ( 'NONE', #13913, #21984, #5704, .T. ) ;
#10239=ORIENTED_EDGE ( 'NONE', *, *, #15059, .F. ) ;
#10265=ORIENTED_EDGE ( 'NONE', *, *, #2473, .F. ) ;
#10269=CARTESIAN_POINT ( 'NONE',  ( 51.99565694909048830, 170.0000000000000284, -0.6720553790413839046 ) ) ;
#10272=EDGE_CURVE ( 'NONE', #7858, #1703, #10372, .T. ) ;
#10273=AXIS2_PLACEMENT_3D ( 'NONE', #7312, #12627, #16420 ) ;
#10274=CARTESIAN_POINT ( 'NONE',  ( -50.94642088777899147, 106.8060942374654871, 71.59769907143252965 ) ) ;
#10284=DIRECTION ( 'NONE',  ( 0.9999164797902017066, 6.965998958219367529E-18, -0.01292414190464157182 ) ) ;
#10298=VECTOR ( 'NONE', #13881, 1000.000000000000000 ) ;
#10303=DIRECTION ( 'NONE',  ( 7.125109674161238737E-05, -0.9999848031710253382, 0.005512562950850163727 ) ) ;
#10316=EDGE_CURVE ( 'NONE', #1571, #9213, #18560, .T. ) ;
#10324=DIRECTION ( 'NONE',  ( 0.9999164797902017066, 6.965998958219365988E-18, -0.01292414190464157356 ) ) ;
#10328=CARTESIAN_POINT ( 'NONE',  ( 14.04531128256715888, 105.6586476617446380, 119.4770396839737714 ) ) ;
#10330=CARTESIAN_POINT ( 'NONE',  ( 18.32483708604867090, 59.11803865240458578, -129.7334415360379580 ) ) ;
#10331=ADVANCED_FACE ( 'NONE', ( #16579 ), #17953, .F. ) ;
#10336=CYLINDRICAL_SURFACE ( 'NONE', #14789, 112.5000000000000142 ) ;
#10338=LINE ( 'NONE', #1607, #14780 ) ;
#10344=EDGE_LOOP ( 'NONE', ( #10775, #13525, #15958, #20905 ) ) ;
#10345=CARTESIAN_POINT ( 'NONE',  ( 50.79682535782767161, 111.7699698251880420, -48.05900560362714202 ) ) ;
#10347=VERTEX_POINT ( 'NONE', #10928 ) ;
#10359=EDGE_CURVE ( 'NONE', #19209, #9134, #9000, .T. ) ;
#10372=LINE ( 'NONE', #11983, #6074 ) ;
#10390=CIRCLE ( 'NONE', #16287, 3.399999999999985700 ) ;
#10395=CARTESIAN_POINT ( 'NONE',  ( -39.99665919160808869, 170.0000000000000284, 0.5169656761856410432 ) ) ;
#10407=CARTESIAN_POINT ( 'NONE',  ( -37.89192165770759146, 95.21750359067902991, 84.54365134533595949 ) ) ;
#10415=CIRCLE ( 'NONE', #9709, 4.199999999999997513 ) ;
#10421=EDGE_LOOP ( 'NONE', ( #801, #16859, #4877, #11211 ) ) ;
#10454=CARTESIAN_POINT ( 'NONE',  ( 50.25207249572593327, 113.2682921568431595, -44.84111833878783671 ) ) ;
#10458=VECTOR ( 'NONE', #721, 1000.000000000000000 ) ;
#10487=ADVANCED_FACE ( 'NONE', ( #21803 ), #4605, .F. ) ;
#10495=VECTOR ( 'NONE', #17025, 1000.000000000000114 ) ;
#10497=EDGE_CURVE ( 'NONE', #22554, #17125, #13118, .T. ) ;
#10498=ORIENTED_EDGE ( 'NONE', *, *, #1773, .F. ) ;
#10499=ADVANCED_FACE ( 'NONE', ( #6205 ), #22028, .F. ) ;
#10500=CARTESIAN_POINT ( 'NONE',  ( -16.77414143088337184, 138.3748544051812246, 249.7078392314084567 ) ) ;
#10509=DIRECTION ( 'NONE',  ( -0.9999164797902015955, -6.965998958219364448E-18, 0.01292414190464157182 ) ) ;
#10520=EDGE_CURVE ( 'NONE', #22544, #14939, #4682, .T. ) ;
#10523=VERTEX_POINT ( 'NONE', #1289 ) ;
#10530=ORIENTED_EDGE ( 'NONE', *, *, #16282, .T. ) ;
#10534=FACE_OUTER_BOUND ( 'NONE', #11071, .T. ) ;
#10536=CARTESIAN_POINT ( 'NONE',  ( 52.02138963284384943, 106.9476250623077789, 70.12004797256865629 ) ) ;
#10541=CARTESIAN_POINT ( 'NONE',  ( -49.99582398951009310, 170.0000000000008242, 0.6462070952329234119 ) ) ;
#10543=CYLINDRICAL_SURFACE ( 'NONE', #11733, 3.399999999999985700 ) ;
#10553=DIRECTION ( 'NONE',  ( 0.9999164797902015955, 6.965998958219364448E-18, -0.01292414190464157182 ) ) ;
#10554=CARTESIAN_POINT ( 'NONE',  ( -48.73516844915841517, 109.8600507193323921, -43.54289476181637042 ) ) ;
#10557=CYLINDRICAL_SURFACE ( 'NONE', #20187, 95.00000000000001421 ) ;
#10565=CARTESIAN_POINT ( 'NONE',  ( 51.53948562937888767, 109.2346207935383120, -44.83551851856461923 ) ) ;
#10566=ORIENTED_EDGE ( 'NONE', *, *, #10085, .F. ) ;
#10573=EDGE_LOOP ( 'NONE', ( #16649, #1610 ) ) ;
#10575=CARTESIAN_POINT ( 'NONE',  ( -45.67488410632294915, 171.6105373975396162, -51.92370490599741117 ) ) ;
#10581=LINE ( 'NONE', #19077, #6312 ) ;
#10605=AXIS2_PLACEMENT_3D ( 'NONE', #4124, #5974, #701 ) ;
#10621=EDGE_CURVE ( 'NONE', #22622, #22296, #8698, .T. ) ;
#10637=CARTESIAN_POINT ( 'NONE',  ( 42.84128820176451313, 101.1708071963161615, 64.81746289747974288 ) ) ;
#10652=CYLINDRICAL_SURFACE ( 'NONE', #4758, 95.00000000000001421 ) ;
#10661=CARTESIAN_POINT ( 'NONE',  ( -40.33104288128404846, 94.48610424851698042, 83.91830964824988826 ) ) ;
#10663=EDGE_LOOP ( 'NONE', ( #11026, #4345, #8401, #3656 ) ) ;
#10665=VECTOR ( 'NONE', #14211, 999.9999999999998863 ) ;
#10681=CARTESIAN_POINT ( 'NONE',  ( -50.56780451594417514, 125.7553391191873544, -43.60684728318641845 ) ) ;
#10685=CARTESIAN_POINT ( 'NONE',  ( -20.57130763759250414, 139.7551263635816952, -44.07174742163757486 ) ) ;
#10695=VECTOR ( 'NONE', #6697, 999.9999999999998863 ) ;
#10696=ORIENTED_EDGE ( 'NONE', *, *, #2370, .T. ) ;
#10697=VERTEX_POINT ( 'NONE', #8477 ) ;
#10701=EDGE_LOOP ( 'NONE', ( #12567, #574, #12509, #14629, #5852, #8380 ) ) ;
#10717=CARTESIAN_POINT ( 'NONE',  ( -29.40402206585522293, 189.4003865961453812, -108.4455932242574789 ) ) ;
#10718=CIRCLE ( 'NONE', #18777, 95.00000000000001421 ) ;
#10721=AXIS2_PLACEMENT_3D ( 'NONE', #1527, #11980, #17258 ) ;
#10727=CIRCLE ( 'NONE', #5943, 110.5324305509042233 ) ;
#10733=CARTESIAN_POINT ( 'NONE',  ( 41.14495236153211977, 95.00650438983588231, -44.60766223544680287 ) ) ;
#10737=CARTESIAN_POINT ( 'NONE',  ( -65.67450334697799974, 189.7102623349352086, -51.76499945731497121 ) ) ;
#10747=ADVANCED_FACE ( 'NONE', ( #17582 ), #15869, .F. ) ;
#10748=VECTOR ( 'NONE', #22041, 1000.000000000000000 ) ;
#10750=FACE_OUTER_BOUND ( 'NONE', #2435, .T. ) ;
#10757=CYLINDRICAL_SURFACE ( 'NONE', #2870, 7.499999999999991118 ) ;
#10759=CIRCLE ( 'NONE', #5981, 3.399999999999985700 ) ;
#10764=DIRECTION ( 'NONE',  ( 7.125109674161246868E-05, -0.9999848031710253382, 0.005512562950850155054 ) ) ;
#10767=EDGE_CURVE ( 'NONE', #17449, #7530, #13079, .T. ) ;
#10768=CARTESIAN_POINT ( 'NONE',  ( 64.99457118636310327, 170.0000000000000284, -0.8400692238017243296 ) ) ;
#10775=ORIENTED_EDGE ( 'NONE', *, *, #4008, .T. ) ;
#10801=CARTESIAN_POINT ( 'NONE',  ( -49.26241605170081073, 111.2512799097718386, -43.54375060610340853 ) ) ;
#10804=CARTESIAN_POINT ( 'NONE',  ( -50.58840307354613941, 96.06212804229784297, -45.20051882889240602 ) ) ;
#10813=CARTESIAN_POINT ( 'NONE',  ( -27.99766143412566421, 170.0000000000008242, 0.3618759733308087312 ) ) ;
#10818=EDGE_LOOP ( 'NONE', ( #427, #9385, #6467, #2963, #16380, #13801, #16482, #8944, #22648, #8661, #9513, #2407, #19706, #15346, #2940, #12020, #2637, #15020, #5590, #11595, #3842, #19788, #5732, #2165 ) ) ;
#10833=EDGE_CURVE ( 'NONE', #8542, #7339, #15477, .T. ) ;
#10865=DIRECTION ( 'NONE',  ( 0.9999164797902015955, 6.965998958219364448E-18, -0.01292414190464157182 ) ) ;
#10877=ADVANCED_FACE ( 'NONE', ( #6395 ), #20613, .T. ) ;
#10897=DIRECTION ( 'NONE',  ( 0.9999164797902015955, 6.965998958219364448E-18, -0.01292414190464157182 ) ) ;
#10906=CARTESIAN_POINT ( 'NONE',  ( 49.99582398951007889, 170.0000000000000284, -0.6462070952321007367 ) ) ;
#10908=CARTESIAN_POINT ( 'NONE',  ( 45.19561618717597185, 127.3639955235004777, 246.9673780573190527 ) ) ;
#10921=ADVANCED_FACE ( 'NONE', ( #8428 ), #15259, .T. ) ;
#10928=CARTESIAN_POINT ( 'NONE',  ( -48.56673365018540522, 108.3817487785542824, -43.53692110109249569 ) ) ;
#10932=ADVANCED_FACE ( 'NONE', ( #8323 ), #6826, .F. ) ;
#10937=FACE_OUTER_BOUND ( 'NONE', #1120, .T. ) ;
#10939=PLANE ( 'NONE',  #3695 ) ;
#10940=DIRECTION ( 'NONE',  ( 0.01292394549866739996, 0.005513023399721131770, 0.9999012842304692006 ) ) ;
#10941=FACE_OUTER_BOUND ( 'NONE', #12522, .T. ) ;
#10958=EDGE_LOOP ( 'NONE', ( #11215, #15595, #5520, #4648 ) ) ;
#10967=DIRECTION ( 'NONE',  ( 0.01292394549866739996, 0.005513023399735009558, 0.9999012842304692006 ) ) ;
#10971=ORIENTED_EDGE ( 'NONE', *, *, #18787, .T. ) ;
#10975=FACE_OUTER_BOUND ( 'NONE', #12318, .T. ) ;
#10992=DIRECTION ( 'NONE',  ( 0.000000000000000000, -0.005512562964840580192, -0.9999848057093461140 ) ) ;
#10999=AXIS2_PLACEMENT_3D ( 'NONE', #2745, #9755, #16769 ) ;
#11007=ORIENTED_EDGE ( 'NONE', *, *, #15459, .F. ) ;
#11015=DIRECTION ( 'NONE',  ( 0.9999164797902015955, 6.965998958219364448E-18, -0.01292414190464157182 ) ) ;
#11018=VECTOR ( 'NONE', #18433, 1000.000000000000000 ) ;
#11019=VECTOR ( 'NONE', #2346, 1000.000000000000114 ) ;
#11025=VECTOR ( 'NONE', #1785, 1000.000000000000000 ) ;
#11026=ORIENTED_EDGE ( 'NONE', *, *, #14305, .F. ) ;
#11027=EDGE_CURVE ( 'NONE', #20773, #3794, #8202, .T. ) ;
#11032=B_SPLINE_CURVE_WITH_KNOTS ( 'NONE', 3,
 ( #7259, #6605, #263, #5407, #5527, #3053, #12446, #12560, #17863, #9082, #8326, #15368, #20618, #11173, #608, #2441 ),
 .UNSPECIFIED., .F., .F.,
 ( 4, 2, 2, 2, 2, 2, 2, 4 ),
 ( -0.003151246785043320189, -0.002357650993505802130, -0.001960853097737045268, -0.001564055201968288624, -0.001167257306199531979, -0.0007704594104307751178, -0.0003736615146620182563, 2.313638110673860507E-05 ),
 .UNSPECIFIED. ) ;
#11040=DIRECTION ( 'NONE',  ( 0.01292394549866738261, 0.005513023399722618428, 0.9999012842304692006 ) ) ;
#11043=CARTESIAN_POINT ( 'NONE',  ( -45.96244189366829858, 171.4878726268958360, -74.17150848012535391 ) ) ;
#11045=EDGE_LOOP ( 'NONE', ( #14579, #11189, #11231, #21664 ) ) ;
#11051=CARTESIAN_POINT ( 'NONE',  ( 50.40347573247742474, 189.6005870223182228, -73.16055181083503101 ) ) ;
#11053=FACE_BOUND ( 'NONE', #6847, .T. ) ;
#11054=DIRECTION ( 'NONE',  ( -0.01292394549866741384, -0.005513023399721131770, -0.9999012842304692006 ) ) ;
#11057=CYLINDRICAL_SURFACE ( 'NONE', #10011, 2.009999999999995346 ) ;
#11059=CARTESIAN_POINT ( 'NONE',  ( 40.48953805856821475, 105.9808811061030553, 91.99283320860411095 ) ) ;
#11068=ADVANCED_FACE ( 'NONE', ( #13054 ), #17018, .T. ) ;
#11069=CIRCLE ( 'NONE', #14766, 3.399999999999985700 ) ;
#11071=EDGE_LOOP ( 'NONE', ( #7012, #3887, #14716, #14163 ) ) ;
#11072=CARTESIAN_POINT ( 'NONE',  ( 40.14615270801867553, 95.25460127842278268, -44.16447546512498690 ) ) ;
#11078=DIRECTION ( 'NONE',  ( -0.01292394549866740863, -0.005513023399721176006, -0.9999012842304692006 ) ) ;
#11082=FACE_OUTER_BOUND ( 'NONE', #19677, .T. ) ;
#11086=AXIS2_PLACEMENT_3D ( 'NONE', #4946, #15551, #14049 ) ;
#11098=CARTESIAN_POINT ( 'NONE',  ( 41.22233984835247611, 119.7725967263615985, 249.0607866758211344 ) ) ;
#11104=DIRECTION ( 'NONE',  ( 7.125109674159588039E-05, -0.9999848031710253382, 0.005512562950848870491 ) ) ;
#11106=DIRECTION ( 'NONE',  ( 0.01292394549866771568, 0.005513023399718815047, 0.9999012842304693116 ) ) ;
#11110=DIRECTION ( 'NONE',  ( 0.9999164797902017066, 6.965998958219365988E-18, -0.01292414190464157356 ) ) ;
#11121=DIRECTION ( 'NONE',  ( -0.009188991635466050092, 0.7031977391749439921, -0.7109349492407662785 ) ) ;
#11131=LINE ( 'NONE', #13096, #18703 ) ;
#11133=AXIS2_PLACEMENT_3D ( 'NONE', #16158, #21399, #12466 ) ;
#11137=CARTESIAN_POINT ( 'NONE',  ( -50.34903424743296796, 95.63295186387540525, -44.50339194506212692 ) ) ;
#11138=ORIENTED_EDGE ( 'NONE', *, *, #4440, .F. ) ;
#11147=DIRECTION ( 'NONE',  ( 0.01292394549866739996, 0.005513023399721131770, 0.9999012842304692006 ) ) ;
#11155=AXIS2_PLACEMENT_3D ( 'NONE', #15398, #9986, #7915 ) ;
#11156=DIRECTION ( 'NONE',  ( -0.01292394549866737220, -0.005513023399721000799, -0.9999012842304692006 ) ) ;
#11163=DIRECTION ( 'NONE',  ( -0.01292394549866739996, -0.005513023399721131770, -0.9999012842304692006 ) ) ;
#11166=CARTESIAN_POINT ( 'NONE',  ( 50.53293774634011726, 189.6008146261148113, -73.12093756438817138 ) ) ;
#11173=CARTESIAN_POINT ( 'NONE',  ( -40.81696164862506038, 106.8158423209496135, 71.47546216999431579 ) ) ;
#11175=DIRECTION ( 'NONE',  ( 0.9999164797902015955, 6.965998958219364448E-18, -0.01292414190464157182 ) ) ;
#11189=ORIENTED_EDGE ( 'NONE', *, *, #7145, .F. ) ;
#11193=AXIS2_PLACEMENT_3D ( 'NONE', #6533, #20763, #3187 ) ;
#11205=EDGE_CURVE ( 'NONE', #17825, #7434, #19917, .T. ) ;
#11208=CARTESIAN_POINT ( 'NONE',  ( -50.56880203129856000, 139.7551263635817236, -43.68402316449832057 ) ) ;
#11211=ORIENTED_EDGE ( 'NONE', *, *, #21203, .F. ) ;
#11214=EDGE_CURVE ( 'NONE', #16088, #2091, #16825, .T. ) ;
#11215=ORIENTED_EDGE ( 'NONE', *, *, #14926, .F. ) ;
#11222=ORIENTED_EDGE ( 'NONE', *, *, #4772, .T. ) ;
#11231=ORIENTED_EDGE ( 'NONE', *, *, #2473, .T. ) ;
#11235=CARTESIAN_POINT ( 'NONE',  ( -34.79726985247908999, 121.2962013336460814, 248.0347590154626971 ) ) ;
#11237=ORIENTED_EDGE ( 'NONE', *, *, #11214, .T. ) ;
#11242=EDGE_CURVE ( 'NONE', #309, #17948, #10150, .T. ) ;
#11248=DIRECTION ( 'NONE',  ( -0.01292394549866704608, -0.005513023399720698957, -0.9999012842304692006 ) ) ;
#11252=( NAMED_UNIT ( * ) SI_UNIT ( $, .STERADIAN. ) SOLID_ANGLE_UNIT ( ) );
#11254=CARTESIAN_POINT ( 'NONE',  ( -40.63773027173701280, 95.80343475218985816, -42.17386218167892764 ) ) ;
#11263=EDGE_CURVE ( 'NONE', #22552, #18970, #20246, .T. ) ;
#11265=CARTESIAN_POINT ( 'NONE',  ( -52.56676294784124792, 113.4816418249608034, -43.51333844217711544 ) ) ;
#11268=DIRECTION ( 'NONE',  ( 7.125109674161246868E-05, -0.9999848031710252272, 0.005512562950850154186 ) ) ;
#11283=CARTESIAN_POINT ( 'NONE',  ( -50.59241450076314806, 108.3707227317548529, -45.51087538574414992 ) ) ;
#11284=VERTEX_POINT ( 'NONE', #3019 ) ;
#11305=FACE_OUTER_BOUND ( 'NONE', #3854, .T. ) ;
#11312=CARTESIAN_POINT ( 'NONE',  ( -36.80549447617401881, 105.5072037373731888, 92.66220808178287882 ) ) ;
#11320=EDGE_CURVE ( 'NONE', #1365, #17586, #7489, .T. ) ;
#11321=CARTESIAN_POINT ( 'NONE',  ( 26.59130080239608418, 189.4003865961453528, -109.1693451709173956 ) ) ;
#11353=DIRECTION ( 'NONE',  ( 7.125109674161246868E-05, -0.9999848031710253382, 0.005512562950850155054 ) ) ;
#11361=EDGE_CURVE ( 'NONE', #20680, #22552, #7031, .T. ) ;
#11371=ADVANCED_FACE ( 'NONE', ( #3475 ), #15670, .T. ) ;
#11375=CARTESIAN_POINT ( 'NONE',  ( -52.78831554946314242, 109.2941709412885700, -43.48738692163240671 ) ) ;
#11376=ORIENTED_EDGE ( 'NONE', *, *, #14777, .T. ) ;
#11383=FACE_OUTER_BOUND ( 'NONE', #13394, .T. ) ;
#11385=DIRECTION ( 'NONE',  ( 0.01292394549866695240, 0.005513023399725255208, 0.9999012842304693116 ) ) ;
#11389=CARTESIAN_POINT ( 'NONE',  ( -38.63026990148117790, 106.6589261331495777, 92.07993625387241821 ) ) ;
#11390=EDGE_CURVE ( 'NONE', #21389, #21004, #13825, .T. ) ;
#11395=ORIENTED_EDGE ( 'NONE', *, *, #8099, .T. ) ;
#11401=TOROIDAL_SURFACE ( 'NONE', #16902, 93.00000000000000000, 2.000000000000000000 ) ;
#11406=CARTESIAN_POINT ( 'NONE',  ( -36.80549447617401881, 105.5072037373731888, 92.66220808178287882 ) ) ;
#11408=DIRECTION ( 'NONE',  ( -0.01292394549866695240, -0.005513023399718316314, -0.9999012842304693116 ) ) ;
#11411=CARTESIAN_POINT ( 'NONE',  ( 49.02652807711002936, 169.5865232450209703, -75.63880341251731920 ) ) ;
#11415=VERTEX_POINT ( 'NONE', #148 ) ;
#11416=CARTESIAN_POINT ( 'NONE',  ( 51.18466195697779142, 140.5066718483590762, 91.33194389089467791 ) ) ;
#11419=DIRECTION ( 'NONE',  ( 7.125109674161259066E-05, -0.9999848031710252272, 0.005512562950850163727 ) ) ;
#11431=ORIENTED_EDGE ( 'NONE', *, *, #7145, .T. ) ;
#11448=DIRECTION ( 'NONE',  ( 0.01292394549866740169, 0.005513023399721270548, 0.9999012842304692006 ) ) ;
#11461=EDGE_LOOP ( 'NONE', ( #4251, #13107, #21103, #12303 ) ) ;
#11466=AXIS2_PLACEMENT_3D ( 'NONE', #5318, #7585, #14199 ) ;
#11469=ADVANCED_FACE ( 'NONE', ( #12101 ), #21043, .F. ) ;
#11479=CARTESIAN_POINT ( 'NONE',  ( -38.92003986412552052, 97.39926864640099780, 83.81297216957182172 ) ) ;
#11484=EDGE_CURVE ( 'NONE', #15391, #15416, #8857, .T. ) ;
#11489=AXIS2_PLACEMENT_3D ( 'NONE', #22224, #10303, #20745 ) ;
#11497=CARTESIAN_POINT ( 'NONE',  ( -49.00853856164501821, 110.7109146754460625, -43.54405268858729983 ) ) ;
#11507=ORIENTED_EDGE ( 'NONE', *, *, #12026, .F. ) ;
#11513=DIRECTION ( 'NONE',  ( -7.125109674161259066E-05, 0.9999848031710252272, -0.005512562950850163727 ) ) ;
#11520=CARTESIAN_POINT ( 'NONE',  ( 49.99582398951009310, 170.0000000000008242, -0.6462070952312342076 ) ) ;
#11521=CARTESIAN_POINT ( 'NONE',  ( -64.99457118636313169, 170.0000000000000284, 0.8400692238016805868 ) ) ;
#11522=ORIENTED_EDGE ( 'NONE', *, *, #15487, .F. ) ;
#11524=AXIS2_PLACEMENT_3D ( 'NONE', #17293, #8223, #12003 ) ;
#11528=EDGE_CURVE ( 'NONE', #719, #309, #11589, .T. ) ;
#11530=CARTESIAN_POINT ( 'NONE',  ( -41.99649215118849810, 170.0000000000000284, 0.5428139599949243221 ) ) ;
#11533=AXIS2_PLACEMENT_3D ( 'NONE', #14176, #21153, #5297 ) ;
#11534=CARTESIAN_POINT ( 'NONE',  ( -49.15102793893406385, 101.1708071963161615, 66.00648395270677327 ) ) ;
#11537=CARTESIAN_POINT ( 'NONE',  ( -37.77863868662843316, 96.04509607205291388, 85.01029411640075750 ) ) ;
#11539=DIRECTION ( 'NONE',  ( -7.125109674161246868E-05, 0.9999848031710253382, -0.005512562950850155054 ) ) ;
#11546=LINE ( 'NONE', #11312, #17303 ) ;
#11550=CARTESIAN_POINT ( 'NONE',  ( -46.77099456471874817, 129.3749911766419700, 250.1451765551053654 ) ) ;
#11558=CARTESIAN_POINT ( 'NONE',  ( -50.99096779290750447, 169.5754971982215125, -76.34619179051411209 ) ) ;
#11561=CARTESIAN_POINT ( 'NONE',  ( -66.42677970909001317, 189.3893605493459233, -109.9672025422466959 ) ) ;
#11570=CARTESIAN_POINT ( 'NONE',  ( 49.56856857351093737, 189.4900557983233398, -93.20024246017386815 ) ) ;
#11585=LINE ( 'NONE', #793, #5117 ) ;
#11589=B_SPLINE_CURVE_WITH_KNOTS ( 'NONE', 3,
 ( #714, #18400, #18287, #11166, #11051, #2322, #16366, #14408, #604, #14521, #12899, #7709, #21372, #2437, #21583, #5989 ),
 .UNSPECIFIED., .F., .F.,
 ( 4, 2, 2, 2, 2, 2, 2, 4 ),
 ( 0.000000000000000000, 0.0003976838443733619953, 0.0007953676887467239906, 0.001193051533120085932, 0.001590735377493447981, 0.002386103066240156251, 0.002783786910613529793, 0.003181470754986902901 ),
 .UNSPECIFIED. ) ;
#11593=AXIS2_PLACEMENT_3D ( 'NONE', #5636, #12672, #12892 ) ;
#11595=ORIENTED_EDGE ( 'NONE', *, *, #5276, .F. ) ;
#11602=CARTESIAN_POINT ( 'NONE',  ( -34.77171180284935303, 125.3750519639578727, 250.0121371040530676 ) ) ;
#11605=EDGE_LOOP ( 'NONE', ( #690, #19662, #11237, #1462 ) ) ;
#11608=DIRECTION ( 'NONE',  ( 0.9999164797902015955, 6.965998958219364448E-18, -0.01292414190464157182 ) ) ;
#11610=CARTESIAN_POINT ( 'NONE',  ( -50.60905219909545849, 112.8337759852537090, -43.53507023493251893 ) ) ;
#11611=VERTEX_POINT ( 'NONE', #6340 ) ;
#11626=CARTESIAN_POINT ( 'NONE',  ( 53.22065341430143803, 129.3749911766419700, 248.8527623646411939 ) ) ;
#11637=DIRECTION ( 'NONE',  ( -7.125109674156763692E-05, 0.9999848031710254492, -0.005512562950846685607 ) ) ;
#11640=DIRECTION ( 'NONE',  ( -0.01292394549866704608, -0.005513023399718946886, -0.9999012842304692006 ) ) ;
#11642=DIRECTION ( 'NONE',  ( 0.9999164797902015955, 6.965998958219364448E-18, -0.01292414190464157182 ) ) ;
#11643=CARTESIAN_POINT ( 'NONE',  ( -51.28019763314280510, 189.4953702477336890, -90.93270303136451105 ) ) ;
#11646=CARTESIAN_POINT ( 'NONE',  ( -64.99457118636313169, 170.0000000000000284, 0.8400692238016805868 ) ) ;
#11654=DIRECTION ( 'NONE',  ( 0.9999164797902015955, 6.965998958219364448E-18, -0.01292414190464157182 ) ) ;
#11659=ORIENTED_EDGE ( 'NONE', *, *, #13656, .F. ) ;
#11660=TOROIDAL_SURFACE ( 'NONE', #7612, 77.00000000000002842, 2.000000000000000000 ) ;
#11664=CARTESIAN_POINT ( 'NONE',  ( -49.49165101955345136, 107.3307887671683432, 70.99333137697747986 ) ) ;
#11672=DIRECTION ( 'NONE',  ( 0.9999164797902017066, 6.965998958219365988E-18, -0.01292414190464157356 ) ) ;
#11674=CARTESIAN_POINT ( 'NONE',  ( -66.42677970909001317, 189.3893605493459233, -109.9672025422466959 ) ) ;
#11696=CARTESIAN_POINT ( 'NONE',  ( -37.16795793340686060, 95.89798883583556233, 85.13463587459933990 ) ) ;
#11706=B_SPLINE_CURVE_WITH_KNOTS ( 'NONE', 3,
 ( #5483, #14595, #21452, #19392, #1825, #5712, #5605, #17820, #12744, #21550, #17924, #21223, #8938, #14246 ),
 .UNSPECIFIED., .F., .F.,
 ( 4, 2, 2, 2, 2, 2, 4 ),
 ( 0.000000000000000000, 0.001153947729383741775, 0.002307895458767483549, 0.002884869323459376012, 0.003461843188151268041, 0.004038817052843160504, 0.004615790917535052967 ),
 .UNSPECIFIED. ) ;
#11712=EDGE_CURVE ( 'NONE', #16304, #18095, #6663, .T. ) ;
#11714=LINE ( 'NONE', #18708, #20285 ) ;
#11715=DIRECTION ( 'NONE',  ( -0.9999164797902017066, -7.033761593999711556E-18, 0.01292414190464155968 ) ) ;
#11717=CARTESIAN_POINT ( 'NONE',  ( 49.99895903776670991, 126.0006686604749291, -0.4036543253946939802 ) ) ;
#11722=CARTESIAN_POINT ( 'NONE',  ( 14.23917046504717021, 105.7413430127404439, 134.4755589474307840 ) ) ;
#11733=AXIS2_PLACEMENT_3D ( 'NONE', #96, #3765, #2043 ) ;
#11735=EDGE_LOOP ( 'NONE', ( #4346, #21722, #10566, #13372 ) ) ;
#11736=CARTESIAN_POINT ( 'NONE',  ( 39.18801548568782067, 107.5071733437152375, 91.66894817112843441 ) ) ;
#11741=AXIS2_PLACEMENT_3D ( 'NONE', #9671, #13357, #946 ) ;
#11753=CARTESIAN_POINT ( 'NONE',  ( -51.99565694909051672, 170.0000000000000284, 0.6720553790413400508 ) ) ;
#11761=FACE_OUTER_BOUND ( 'NONE', #7670, .T. ) ;
#11765=AXIS2_PLACEMENT_3D ( 'NONE', #774, #18235, #11448 ) ;
#11776=CARTESIAN_POINT ( 'NONE',  ( -21.61166911467453389, 64.93155780410928912, -124.5625524242976070 ) ) ;
#11782=EDGE_CURVE ( 'NONE', #10176, #7226, #7126, .T. ) ;
#11786=B_SPLINE_CURVE_WITH_KNOTS ( 'NONE', 3,
 ( #21784, #16223, #6075, #3991, #12862, #18366, #7574, #19841, #7461, #16340, #12993, #11254, #13104, #14499, #21460, #18045 ),
 .UNSPECIFIED., .F., .F.,
 ( 4, 2, 2, 2, 2, 2, 2, 4 ),
 ( 6.938893903907228378E-18, 0.0004210512469646337250, 0.0008421024939292605111, 0.001684204987858477871, 0.002105256234823093056, 0.002526307481787708024, 0.002947358728752323426, 0.003368409975716938395 ),
 .UNSPECIFIED. ) ;
#11788=EDGE_CURVE ( 'NONE', #2512, #16435, #1832, .T. ) ;
#11796=CIRCLE ( 'NONE', #14749, 95.00000000000001421 ) ;
#11798=ORIENTED_EDGE ( 'NONE', *, *, #12048, .T. ) ;
#11800=ORIENTED_EDGE ( 'NONE', *, *, #17285, .F. ) ;
#11809=AXIS2_PLACEMENT_3D ( 'NONE', #20097, #11513, #18076 ) ;
#11812=ORIENTED_EDGE ( 'NONE', *, *, #11788, .T. ) ;
#11824=LINE ( 'NONE', #18814, #21059 ) ;
#11834=DIRECTION ( 'NONE',  ( 0.01292394549866740863, 0.005513023399721176006, 0.9999012842304692006 ) ) ;
#11835=VECTOR ( 'NONE', #1712, 1000.000000000000114 ) ;
#11849=CARTESIAN_POINT ( 'NONE',  ( 50.67479067645616198, 109.8916839534814471, -44.82796490703182712 ) ) ;
#11850=ORIENTED_EDGE ( 'NONE', *, *, #17235, .F. ) ;
#11852=CARTESIAN_POINT ( 'NONE',  ( -39.99338164115797412, 124.0006990541328804, 0.7705435719247482051 ) ) ;
#11859=LINE ( 'NONE', #18524, #3600 ) ;
#11860=CARTESIAN_POINT ( 'NONE',  ( 49.99582398951007889, 170.0000000000000284, -0.6462070952321007367 ) ) ;
#11873=CARTESIAN_POINT ( 'NONE',  ( 50.81961426468491538, 113.4359159616137731, -44.84937814700944614 ) ) ;
#11881=DIRECTION ( 'NONE',  ( 0.01292394549866738261, 0.005513023399722618428, 0.9999012842304692006 ) ) ;
#11891=VERTEX_POINT ( 'NONE', #10908 ) ;
#11895=VECTOR ( 'NONE', #11539, 999.9999999999998863 ) ;
#11904=EDGE_CURVE ( 'NONE', #18552, #12549, #18151, .T. ) ;
#11909=CARTESIAN_POINT ( 'NONE',  ( -51.14300816381444292, 189.5947554187170851, -72.90590013953031701 ) ) ;
#11914=VECTOR ( 'NONE', #14946, 1000.000000000000000 ) ;
#11918=CYLINDRICAL_SURFACE ( 'NONE', #13618, 1.999999999999998446 ) ;
#11924=VECTOR ( 'NONE', #6592, 1000.000000000000000 ) ;
#11932=EDGE_CURVE ( 'NONE', #1664, #3576, #2361, .T. ) ;
#11934=CARTESIAN_POINT ( 'NONE',  ( -10.90995169204228610, 105.6768406389637107, 123.0998174695503451 ) ) ;
#11945=FACE_OUTER_BOUND ( 'NONE', #14635, .T. ) ;
#11950=EDGE_CURVE ( 'NONE', #18464, #3864, #9166, .T. ) ;
#11952=DIRECTION ( 'NONE',  ( -0.9999164797902015955, -6.965998958219364448E-18, 0.01292414190464157182 ) ) ;
#11954=ORIENTED_EDGE ( 'NONE', *, *, #14453, .F. ) ;
#11960=CARTESIAN_POINT ( 'NONE',  ( 51.76191778456981751, 109.4814342785208368, -44.83975432626324675 ) ) ;
#11964=CARTESIAN_POINT ( 'NONE',  ( -27.02995630134907046, 99.74539563421257071, 75.23139667190513080 ) ) ;
#11969=CARTESIAN_POINT ( 'NONE',  ( 48.80621279012751046, 95.32702374722853733, -45.27713056539194270 ) ) ;
#11971=FACE_OUTER_BOUND ( 'NONE', #9769, .T. ) ;
#11977=ORIENTED_EDGE ( 'NONE', *, *, #13839, .T. ) ;
#11978=ORIENTED_EDGE ( 'NONE', *, *, #19106, .F. ) ;
#11980=DIRECTION ( 'NONE',  ( 7.125109674159586684E-05, -0.9999848031710252272, 0.005512562950848869624 ) ) ;
#11983=CARTESIAN_POINT ( 'NONE',  ( -61.79544715037562241, 127.3639955235004777, 248.3502612411157315 ) ) ;
#11986=ORIENTED_EDGE ( 'NONE', *, *, #22220, .F. ) ;
#11989=DIRECTION ( 'NONE',  ( 0.9999164797902015955, 6.965998958219364448E-18, -0.01292414190464157182 ) ) ;
#11990=CYLINDRICAL_SURFACE ( 'NONE', #14761, 4.199999999999997513 ) ;
#12003=DIRECTION ( 'NONE',  ( -0.01292394549866744159, -0.005513023399721009472, -0.9999012842304692006 ) ) ;
#12010=DIRECTION ( 'NONE',  ( 0.9999164797902017066, 6.965998958219365988E-18, -0.01292414190464157356 ) ) ;
#12012=DIRECTION ( 'NONE',  ( 0.01292394549866743812, 0.005513023399720639109, 0.9999012842304693116 ) ) ;
#12014=CIRCLE ( 'NONE', #17519, 112.5000000000000142 ) ;
#12020=ORIENTED_EDGE ( 'NONE', *, *, #7097, .T. ) ;
#12026=EDGE_CURVE ( 'NONE', #1318, #2070, #12698, .T. ) ;
#12037=AXIS2_PLACEMENT_3D ( 'NONE', #11520, #2996, #22046 ) ;
#12040=DIRECTION ( 'NONE',  ( 7.125109674161259066E-05, -0.9999848031710252272, 0.005512562950850163727 ) ) ;
#12048=EDGE_CURVE ( 'NONE', #14615, #11284, #7909, .T. ) ;
#12058=AXIS2_PLACEMENT_3D ( 'NONE', #7482, #5740, #9420 ) ;
#12059=AXIS2_PLACEMENT_3D ( 'NONE', #1307, #4823, #961 ) ;
#12064=CARTESIAN_POINT ( 'NONE',  ( -51.54031057290245599, 113.3115871737369673, -43.52566795857408266 ) ) ;
#12066=EDGE_CURVE ( 'NONE', #7339, #2719, #11824, .T. ) ;
#12067=CARTESIAN_POINT ( 'NONE',  ( 51.66853286597432771, 109.8098455164457619, -44.84035802310724250 ) ) ;
#12069=DIRECTION ( 'NONE',  ( 0.000000000000000000, 0.000000000000000000, 1.000000000000000000 ) ) ;
#12087=LINE ( 'NONE', #8393, #5570 ) ;
#12093=DIRECTION ( 'NONE',  ( -7.125109674161230605E-05, 0.9999848031710253382, -0.005512562950850140309 ) ) ;
#12101=FACE_OUTER_BOUND ( 'NONE', #7285, .T. ) ;
#12102=DIRECTION ( 'NONE',  ( -0.01292394549866704608, -0.005513023399720698957, -0.9999012842304692006 ) ) ;
#12103=CARTESIAN_POINT ( 'NONE',  ( 40.57355171551004247, 108.0982075334647163, 198.8652726751216733 ) ) ;
#12109=EDGE_LOOP ( 'NONE', ( #21462, #20082, #9807, #5731 ) ) ;
#12110=AXIS2_PLACEMENT_3D ( 'NONE', #12750, #14600, #18040 ) ;
#12111=EDGE_LOOP ( 'NONE', ( #21039, #8918, #13150, #10971, #2571, #8052, #19191, #5216, #7144, #22269 ) ) ;
#12117=LINE ( 'NONE', #13949, #15377 ) ;
#12131=CARTESIAN_POINT ( 'NONE',  ( 41.42451162475439475, 125.7553391191873544, -44.79586833841344173 ) ) ;
#12139=AXIS2_PLACEMENT_3D ( 'NONE', #1494, #15521, #22471 ) ;
#12144=VECTOR ( 'NONE', #14903, 1000.000000000000114 ) ;
#12147=ORIENTED_EDGE ( 'NONE', *, *, #3881, .F. ) ;
#12148=CARTESIAN_POINT ( 'NONE',  ( 64.02527527396304663, 169.5865232450209703, -75.83266554108695345 ) ) ;
#12149=EDGE_CURVE ( 'NONE', #1745, #17283, #8575, .T. ) ;
#12158=PRODUCT_DEFINITION_SHAPE ( 'NONE', 'NONE',  #1029 ) ;
#12170=EDGE_CURVE ( 'NONE', #18473, #20719, #1639, .T. ) ;
#12176=CARTESIAN_POINT ( 'NONE',  ( -48.56675489936627343, 108.6799603325455763, -43.53856503602677464 ) ) ;
#12187=CARTESIAN_POINT ( 'NONE',  ( 48.60502302639385874, 111.9953525209499645, -44.81281142087428293 ) ) ;
#12189=VERTEX_POINT ( 'NONE', #20644 ) ;
#12195=CARTESIAN_POINT ( 'NONE',  ( 49.99582398951007889, 170.0000000000000284, -0.6462070952321007367 ) ) ;
#12214=CIRCLE ( 'NONE', #2298, 9.921742784567037177 ) ;
#12217=CARTESIAN_POINT ( 'NONE',  ( 64.31563894222803413, 189.7102623349352086, -53.44515082906027459 ) ) ;
#12218=ORIENTED_EDGE ( 'NONE', *, *, #21684, .T. ) ;
#12226=AXIS2_PLACEMENT_3D ( 'NONE', #7326, #14370, #570 ) ;
#12237=DIRECTION ( 'NONE',  ( 7.125109674161246868E-05, -0.9999848031710253382, 0.005512562950850155054 ) ) ;
#12241=CARTESIAN_POINT ( 'NONE',  ( -38.93830720113543009, 95.97017003981163441, 82.39966276358782693 ) ) ;
#12247=VECTOR ( 'NONE', #21522, 999.9999999999998863 ) ;
#12248=CARTESIAN_POINT ( 'NONE',  ( 14.23917046504717021, 105.7413430127404439, 134.4755589474307840 ) ) ;
#12250=CARTESIAN_POINT ( 'NONE',  ( -36.90283430563165723, 95.89798883583559075, 85.13120909300619132 ) ) ;
#12251=FACE_OUTER_BOUND ( 'NONE', #21159, .T. ) ;
#12255=ORIENTED_EDGE ( 'NONE', *, *, #17979, .T. ) ;
#12278=CIRCLE ( 'NONE', #3077, 4.199999999999997513 ) ;
#12279=ORIENTED_EDGE ( 'NONE', *, *, #7267, .F. ) ;
#12290=AXIS2_PLACEMENT_3D ( 'NONE', #21458, #2167, #16339 ) ;
#12294=DIRECTION ( 'NONE',  ( 0.01292394549866695240, 0.005513023399718316314, 0.9999012842304693116 ) ) ;
#12295=LINE ( 'NONE', #19273, #5200 ) ;
#12297=AXIS2_PLACEMENT_3D ( 'NONE', #10106, #2973, #4674 ) ;
#12300=DIRECTION ( 'NONE',  ( 0.9999164797902017066, 6.965998958219365988E-18, -0.01292414190464157356 ) ) ;
#12303=ORIENTED_EDGE ( 'NONE', *, *, #2852, .F. ) ;
#12308=CARTESIAN_POINT ( 'NONE',  ( 48.12047892932057636, 111.2511799747316559, -44.80244553543491293 ) ) ;
#12312=CIRCLE ( 'NONE', #563, 2.000000000000001332 ) ;
#12315=EDGE_CURVE ( 'NONE', #20578, #13213, #16075, .T. ) ;
#12316=DIRECTION ( 'NONE',  ( -0.01292394549866739996, -0.005513023399721131770, -0.9999012842304692006 ) ) ;
#12318=EDGE_LOOP ( 'NONE', ( #19912, #17404, #17900, #22389, #9254, #2578 ) ) ;
#12320=FACE_OUTER_BOUND ( 'NONE', #21078, .T. ) ;
#12323=CARTESIAN_POINT ( 'NONE',  ( -51.42433909778522150, 169.3906321239456361, -109.8753121617313724 ) ) ;
#12328=CARTESIAN_POINT ( 'NONE',  ( -34.79726985247908999, 121.2962013336460814, 248.0347590154626971 ) ) ;
#12329=CARTESIAN_POINT ( 'NONE',  ( -51.19775092088617185, 169.4872888238259634, -92.34461233820157133 ) ) ;
#12332=CARTESIAN_POINT ( 'NONE',  ( -64.99457118636311748, 170.0000000000008242, 0.8400692238025471159 ) ) ;
#12334=ORIENTED_EDGE ( 'NONE', *, *, #19870, .T. ) ;
#12342=CARTESIAN_POINT ( 'NONE',  ( 68.19355272015712899, 129.3639651298425406, 246.6590976676106095 ) ) ;
#12346=ORIENTED_EDGE ( 'NONE', *, *, #13604, .T. ) ;
#12350=ORIENTED_EDGE ( 'NONE', *, *, #17659, .T. ) ;
#12351=ORIENTED_EDGE ( 'NONE', *, *, #19091, .T. ) ;
#12356=DIRECTION ( 'NONE',  ( 0.01292394549866738261, 0.005513023399721051106, 0.9999012842304692006 ) ) ;
#12359=CARTESIAN_POINT ( 'NONE',  ( -40.72903392649028120, 95.05466328596200754, 83.34854290912163322 ) ) ;
#12361=ORIENTED_EDGE ( 'NONE', *, *, #16268, .F. ) ;
#12371=DIRECTION ( 'NONE',  ( -7.125109674141484573E-05, 0.9999848031710252272, -0.005512562950865663482 ) ) ;
#12374=VERTEX_POINT ( 'NONE', #9739 ) ;
#12394=CARTESIAN_POINT ( 'NONE',  ( -51.44976785811018516, 169.3797848675314128, -111.8426873806957502 ) ) ;
#12395=CARTESIAN_POINT ( 'NONE',  ( -49.99582398951010731, 170.0000000000000284, 0.6462070952320568828 ) ) ;
#12396=CARTESIAN_POINT ( 'NONE',  ( -20.57130763759250414, 139.7551263635816952, -44.07174742163757486 ) ) ;
#12402=ORIENTED_EDGE ( 'NONE', *, *, #3358, .F. ) ;
#12405=CARTESIAN_POINT ( 'NONE',  ( 49.99582398951007889, 170.0000000000000284, -0.6462070952321007367 ) ) ;
#12407=CIRCLE ( 'NONE', #1032, 102.6746853779045381 ) ;
#12416=CARTESIAN_POINT ( 'NONE',  ( -49.99582398951009310, 170.0000000000008242, 0.6462070952329234119 ) ) ;
#12422=FACE_OUTER_BOUND ( 'NONE', #19703, .T. ) ;
#12428=CARTESIAN_POINT ( 'NONE',  ( 64.99457118636310327, 170.0000000000000284, -0.8400692238017243296 ) ) ;
#12433=FACE_BOUND ( 'NONE', #5539, .T. ) ;
#12438=CARTESIAN_POINT ( 'NONE',  ( -63.91682626075579066, 94.48610424851698042, 84.22316112083726125 ) ) ;
#12446=CARTESIAN_POINT ( 'NONE',  ( -39.56633482716346606, 107.3157093434689244, 71.90145589903634971 ) ) ;
#12447=SURFACE_SIDE_STYLE ('',( #5408 ) ) ;
#12449=DIRECTION ( 'NONE',  ( 0.9999164797902017066, 6.965998958219365988E-18, -0.01292414190464157356 ) ) ;
#12462=DIRECTION ( 'NONE',  ( 0.01292394549866740169, 0.005513023399720822990, 0.9999012842304693116 ) ) ;
#12466=DIRECTION ( 'NONE',  ( 0.01292394549866737741, 0.005513023399721125699, 0.9999012842304693116 ) ) ;
#12498=AXIS2_PLACEMENT_3D ( 'NONE', #12853, #9638, #911 ) ;
#12501=ORIENTED_EDGE ( 'NONE', *, *, #18824, .F. ) ;
#12508=VECTOR ( 'NONE', #18223, 1000.000000000000114 ) ;
#12509=ORIENTED_EDGE ( 'NONE', *, *, #511, .T. ) ;
#12511=ADVANCED_FACE ( 'NONE', ( #21160 ), #374, .T. ) ;
#12517=ORIENTED_EDGE ( 'NONE', *, *, #17659, .F. ) ;
#12522=EDGE_LOOP ( 'NONE', ( #12218, #18623, #15821, #2685 ) ) ;
#12544=CARTESIAN_POINT ( 'NONE',  ( -65.60787997720018438, 111.9218655255082382, -46.61047501217030486 ) ) ;
#12549=VERTEX_POINT ( 'NONE', #7154 ) ;
#12551=EDGE_LOOP ( 'NONE', ( #20533, #18325, #20012, #8770, #21821, #3316 ) ) ;
#12556=AXIS2_PLACEMENT_3D ( 'NONE', #11964, #18946, #17132 ) ;
#12560=CARTESIAN_POINT ( 'NONE',  ( -39.75239154531121955, 107.1767517790489705, 71.78158818304505928 ) ) ;
#12562=CARTESIAN_POINT ( 'NONE',  ( -41.22219898879972533, 106.9149828242082947, 60.44841535108972153 ) ) ;
#12563=EDGE_LOOP ( 'NONE', ( #17380, #18978, #15565, #9882 ) ) ;
#12565=AXIS2_PLACEMENT_3D ( 'NONE', #3907, #14169, #21145 ) ;
#12567=ORIENTED_EDGE ( 'NONE', *, *, #18216, .F. ) ;
#12569=ORIENTED_EDGE ( 'NONE', *, *, #14699, .F. ) ;
#12570=FACE_OUTER_BOUND ( 'NONE', #269, .T. ) ;
#12573=EDGE_CURVE ( 'NONE', #6559, #883, #11032, .T. ) ;
#12576=CIRCLE ( 'NONE', #22329, 7.921742784567035400 ) ;
#12581=CARTESIAN_POINT ( 'NONE',  ( -38.86688258710752564, 95.50318961173329058, 82.87093702155239328 ) ) ;
#12591=AXIS2_PLACEMENT_3D ( 'NONE', #8814, #15864, #109 ) ;
#12594=CARTESIAN_POINT ( 'NONE',  ( -39.06279898716250187, 108.3240682923980245, 72.76796811295301382 ) ) ;
#12595=CARTESIAN_POINT ( 'NONE',  ( -21.30129866354426582, 189.4444907833431273, -100.5497760856508478 ) ) ;
#12606=ADVANCED_FACE ( 'NONE', ( #13130 ), #11057, .F. ) ;
#12619=AXIS2_PLACEMENT_3D ( 'NONE', #16276, #18430, #19901 ) ;
#12620=ADVANCED_FACE ( 'NONE', ( #4365 ), #5995, .T. ) ;
#12625=ADVANCED_FACE ( 'NONE', ( #21488 ), #19992, .T. ) ;
#12627=DIRECTION ( 'NONE',  ( -7.125109674158749138E-05, 0.9999848031710253382, -0.005512562950850162860 ) ) ;
#12644=CIRCLE ( 'NONE', #7113, 2.000000000000001332 ) ;
#12645=FACE_OUTER_BOUND ( 'NONE', #2274, .T. ) ;
#12646=CARTESIAN_POINT ( 'NONE',  ( -48.56578001921132426, 94.99786382055523859, -43.46314047150291060 ) ) ;
#12658=CARTESIAN_POINT ( 'NONE',  ( 41.09169241204631362, 95.99012513974443550, 84.20368898025243709 ) ) ;
#12667=ORIENTED_EDGE ( 'NONE', *, *, #11904, .T. ) ;
#12672=DIRECTION ( 'NONE',  ( -0.01292394549866740169, -0.005513023399719838534, -0.9999012842304693116 ) ) ;
#12681=DIRECTION ( 'NONE',  ( 0.01292394549866739996, 0.005513023399721131770, 0.9999012842304692006 ) ) ;
#12687=ORIENTED_EDGE ( 'NONE', *, *, #12573, .F. ) ;
#12698=B_SPLINE_CURVE_WITH_KNOTS ( 'NONE', 3,
 ( #11479, #20070, #9757, #18364, #6307, #4454, #13211, #13332, #20518, #4564, #2634, #13436, #11696, #17003 ),
 .UNSPECIFIED., .F., .F.,
 ( 4, 2, 2, 2, 2, 2, 4 ),
 ( 1.387778780781445676E-17, 0.0003920573607328231873, 0.0007841147214656324967, 0.001176172082198441698, 0.001568229442931251116, 0.002352344164396850002, 0.003136458885862449322 ),
 .UNSPECIFIED. ) ;
#12700=CARTESIAN_POINT ( 'NONE',  ( 27.99766143412564290, 170.0000000000008242, -0.3618759733291194713 ) ) ;
#12705=EDGE_CURVE ( 'NONE', #19209, #6360, #2879, .T. ) ;
#12708=SHAPE_REPRESENTATION_RELATIONSHIP ( 'NONE' , 'NONE' ,  #2270, #19482 ) ;
#12713=ORIENTED_EDGE ( 'NONE', *, *, #17873, .F. ) ;
#12714=LINE ( 'NONE', #19682, #13971 ) ;
#12726=CARTESIAN_POINT ( 'NONE',  ( 66.07231611197045140, 94.48610424851698042, 82.54302267323386388 ) ) ;
#12735=VERTEX_POINT ( 'NONE', #20443 ) ;
#12742=DIRECTION ( 'NONE',  ( -7.125109674161231961E-05, 0.9999848031710252272, -0.005512562950850142043 ) ) ;
#12744=CARTESIAN_POINT ( 'NONE',  ( 50.25511493332505353, 111.2913824189418364, -47.87582765672370044 ) ) ;
#12746=ORIENTED_EDGE ( 'NONE', *, *, #20555, .F. ) ;
#12747=CARTESIAN_POINT ( 'NONE',  ( 42.91324393340197219, 106.8060942374655156, 70.38454212103849272 ) ) ;
#12748=CARTESIAN_POINT ( 'NONE',  ( 50.76788212671708322, 169.4762627770265340, -95.66267738093596051 ) ) ;
#12750=CARTESIAN_POINT ( 'NONE',  ( -41.94323954856972136, 174.9483409995870886, 5.436613131876677940 ) ) ;
#12756=EDGE_CURVE ( 'NONE', #21685, #2070, #124, .T. ) ;
#12761=CARTESIAN_POINT ( 'NONE',  ( 41.12451612944703783, 107.6443775000873160, 71.14585205175409044 ) ) ;
#12777=DIRECTION ( 'NONE',  ( 0.009188991635466048358, -0.7031977391749438810, 0.7109349492407661675 ) ) ;
#12783=DIRECTION ( 'NONE',  ( 0.01292394549866695240, 0.005513023399711377420, 0.9999012842304693116 ) ) ;
#12784=CARTESIAN_POINT ( 'NONE',  ( 40.58925859504437739, 106.0715746962035695, 92.05426835618892767 ) ) ;
#12785=AXIS2_PLACEMENT_3D ( 'NONE', #11736, #2883, #8495 ) ;
#12794=ORIENTED_EDGE ( 'NONE', *, *, #15823, .F. ) ;
#12797=EDGE_CURVE ( 'NONE', #4876, #13067, #17591, .T. ) ;
#12798=CARTESIAN_POINT ( 'NONE',  ( 39.62116574264821622, 95.66828032177839702, -43.44368198931868363 ) ) ;
#12799=DIRECTION ( 'NONE',  ( 0.01292394549866737567, 0.005513023399721124831, 0.9999012842304693116 ) ) ;
#12814=CIRCLE ( 'NONE', #22318, 2.000000000000001332 ) ;
#12818=AXIS2_PLACEMENT_3D ( 'NONE', #1711, #3301, #12294 ) ;
#12821=CARTESIAN_POINT ( 'NONE',  ( 26.28163433660693471, 55.00725983767637928, -133.1276554916787518 ) ) ;
#12824=CARTESIAN_POINT ( 'NONE',  ( 41.22179815901248645, 127.3750215702999213, 249.0188771933985663 ) ) ;
#12825=LINE ( 'NONE', #19804, #6375 ) ;
#12826=ORIENTED_EDGE ( 'NONE', *, *, #17818, .T. ) ;
#12847=EDGE_CURVE ( 'NONE', #3054, #8988, #1238, .T. ) ;
#12853=CARTESIAN_POINT ( 'NONE',  ( -27.99766143412566421, 170.0000000000008242, 0.3618759733308087312 ) ) ;
#12856=CARTESIAN_POINT ( 'NONE',  ( 40.57709715711068554, 106.0996895337223265, 199.1395768038429424 ) ) ;
#12862=CARTESIAN_POINT ( 'NONE',  ( -41.87517931370788915, 95.06543052087248213, -43.43230847621652657 ) ) ;
#12864=AXIS2_PLACEMENT_3D ( 'NONE', #15482, #4985, #12012 ) ;
#12866=EDGE_CURVE ( 'NONE', #13585, #21883, #10759, .T. ) ;
#12868=AXIS2_PLACEMENT_3D ( 'NONE', #12328, #140, #7138 ) ;
#12874=CARTESIAN_POINT ( 'NONE',  ( 41.41151635295819489, 107.3156853856626043, 70.85477822274174287 ) ) ;
#12883=ADVANCED_FACE ( 'NONE', ( #3, #14034, #14259 ), #21132, .F. ) ;
#12886=ORIENTED_EDGE ( 'NONE', *, *, #19241, .T. ) ;
#12889=DIRECTION ( 'NONE',  ( -0.01292394549866739996, -0.005513023399721131770, -0.9999012842304692006 ) ) ;
#12892=DIRECTION ( 'NONE',  ( 7.125109674159588039E-05, -0.9999848031710253382, 0.005512562950848870491 ) ) ;
#12898=VECTOR ( 'NONE', #5146, 1000.000000000000114 ) ;
#12899=CARTESIAN_POINT ( 'NONE',  ( 49.29218688498771428, 189.5954397161826535, -74.07991498343932335 ) ) ;
#12902=EDGE_CURVE ( 'NONE', #3576, #3054, #1593, .T. ) ;
#12905=CARTESIAN_POINT ( 'NONE',  ( 45.19547368498248829, 129.3639651298425406, 246.9563529314173707 ) ) ;
#12906=B_SPLINE_CURVE_WITH_KNOTS ( 'NONE', 3,
 ( #12646, #15990, #1953, #3781, #21228, #7455, #19513, #9396, #119, #7117, #2164, #11137, #9163, #16217, #10804, #338 ),
 .UNSPECIFIED., .F., .F.,
 ( 4, 2, 2, 2, 2, 2, 2, 4 ),
 ( 6.938893903907227607E-18, 0.0004255381963929606411, 0.0008510763927859143433, 0.001276614589178868154, 0.001702152785571821748, 0.002127690981964775775, 0.002553229178357729369, 0.003404305571143620077 ),
 .UNSPECIFIED. ) ;
#12912=EDGE_CURVE ( 'NONE', #9625, #16088, #4871, .T. ) ;
#12925=CARTESIAN_POINT ( 'NONE',  ( -45.96219963993937796, 168.0879242961143518, -74.15276576609245751 ) ) ;
#12930=DIRECTION ( 'NONE',  ( 0.9999164797902015955, 6.965998958219364448E-18, -0.01292414190464157182 ) ) ;
#12935=CARTESIAN_POINT ( 'NONE',  ( -38.79722561300751238, 125.3640259171584290, 248.0640311032106524 ) ) ;
#12947=CIRCLE ( 'NONE', #6688, 2.000000000000001332 ) ;
#12949=CARTESIAN_POINT ( 'NONE',  ( -29.71368853164436530, 55.00725983767640770, -132.4039035450188351 ) ) ;
#12950=ORIENTED_EDGE ( 'NONE', *, *, #19618, .F. ) ;
#12962=AXIS2_PLACEMENT_3D ( 'NONE', #6218, #19653, #10940 ) ;
#12966=CARTESIAN_POINT ( 'NONE',  ( 44.03028354117878251, 168.0879242961143518, -75.31593853751020617 ) ) ;
#12983=DIRECTION ( 'NONE',  ( -7.125109674159588039E-05, 0.9999848031710253382, -0.005512562950848870491 ) ) ;
#12986=VECTOR ( 'NONE', #22092, 999.9999999999998863 ) ;
#12988=CARTESIAN_POINT ( 'NONE',  ( -41.07974036897499559, 106.8060942374655156, 71.47017004102838200 ) ) ;
#12993=CARTESIAN_POINT ( 'NONE',  ( -40.73077958905026463, 95.66828137409537192, -42.40511349254944662 ) ) ;
#12997=AXIS2_PLACEMENT_3D ( 'NONE', #16744, #2596, #16510 ) ;
#13005=CARTESIAN_POINT ( 'NONE',  ( 40.97829051141438583, 107.9174786211642214, 71.38475741957512355 ) ) ;
#13008=VECTOR ( 'NONE', #20856, 1000.000000000000000 ) ;
#13009=ORIENTED_EDGE ( 'NONE', *, *, #12902, .F. ) ;
#13013=EDGE_CURVE ( 'NONE', #22296, #7530, #14445, .T. ) ;
#13014=CARTESIAN_POINT ( 'NONE',  ( -52.71146364212827962, 109.8959631047793124, -43.49169827137859556 ) ) ;
#13016=VERTEX_POINT ( 'NONE', #8130 ) ;
#13022=VERTEX_POINT ( 'NONE', #3274 ) ;
#13033=CARTESIAN_POINT ( 'NONE',  ( 50.77011715189885166, 106.9149828242082947, 59.25939429586269824 ) ) ;
#13034=CIRCLE ( 'NONE', #20703, 102.6746853779045381 ) ;
#13041=ORIENTED_EDGE ( 'NONE', *, *, #8919, .T. ) ;
#13049=DIRECTION ( 'NONE',  ( -0.01292394549866695240, -0.005513023399718316314, -0.9999012842304693116 ) ) ;
#13054=FACE_OUTER_BOUND ( 'NONE', #1625, .T. ) ;
#13061=EDGE_CURVE ( 'NONE', #2491, #15391, #3051, .T. ) ;
#13067=VERTEX_POINT ( 'NONE', #19250 ) ;
#13070=DIRECTION ( 'NONE',  ( 0.9999164797902015955, 6.965998958219364448E-18, -0.01292414190464157182 ) ) ;
#13077=DIRECTION ( 'NONE',  ( -0.01292394549866739996, -0.005513023399721131770, -0.9999012842304692006 ) ) ;
#13079=LINE ( 'NONE', #335, #18119 ) ;
#13080=DIRECTION ( 'NONE',  ( 0.9999164797902015955, 6.965998958219364448E-18, -0.01292414190464157182 ) ) ;
#13089=VECTOR ( 'NONE', #8368, 1000.000000000000000 ) ;
#13091=FACE_BOUND ( 'NONE', #13452, .T. ) ;
#13094=EDGE_CURVE ( 'NONE', #17125, #163, #10390, .T. ) ;
#13096=CARTESIAN_POINT ( 'NONE',  ( -46.77031037318527495, 119.7725967263615985, 250.1981111634296155 ) ) ;
#13104=CARTESIAN_POINT ( 'NONE',  ( -40.60272855283507454, 95.87258248339890088, -42.05554350543408759 ) ) ;
#13107=ORIENTED_EDGE ( 'NONE', *, *, #881, .F. ) ;
#13112=CARTESIAN_POINT ( 'NONE',  ( 48.76804916713667382, 169.4762627770265340, -95.63682909712669300 ) ) ;
#13117=CARTESIAN_POINT ( 'NONE',  ( 51.99565694909048830, 170.0000000000000284, -0.6720553790413839046 ) ) ;
#13118=LINE ( 'NONE', #13560, #590 ) ;
#13124=CARTESIAN_POINT ( 'NONE',  ( 14.08568026761702896, 137.6763543404365180, 122.6003119075071197 ) ) ;
#13127=FACE_OUTER_BOUND ( 'NONE', #19192, .T. ) ;
#13130=FACE_OUTER_BOUND ( 'NONE', #10663, .T. ) ;
#13132=CARTESIAN_POINT ( 'NONE',  ( -51.88145199138811137, 111.6854492628015976, -46.70071095239993042 ) ) ;
#13142=CARTESIAN_POINT ( 'NONE',  ( -37.35473898174801377, 105.5788163333585743, 92.63175017747209949 ) ) ;
#13150=ORIENTED_EDGE ( 'NONE', *, *, #17235, .T. ) ;
#13152=DIRECTION ( 'NONE',  ( -0.01292394549866740863, -0.005513023399721009472, -0.9999012842304692006 ) ) ;
#13165=VERTEX_POINT ( 'NONE', #3744 ) ;
#13166=DIRECTION ( 'NONE',  ( 0.01292394549866705648, 0.005513023399720703294, 0.9999012842304692006 ) ) ;
#13178=EDGE_CURVE ( 'NONE', #21686, #6519, #4516, .T. ) ;
#13182=DIRECTION ( 'NONE',  ( 0.01292394549866739996, 0.005513023399721131770, 0.9999012842304692006 ) ) ;
#13183=CARTESIAN_POINT ( 'NONE',  ( -40.07963149416921311, 107.0053247559780090, 71.63428818222637062 ) ) ;
#13189=VECTOR ( 'NONE', #14539, 1000.000000000000000 ) ;
#13196=EDGE_CURVE ( 'NONE', #19195, #4059, #887, .T. ) ;
#13201=ADVANCED_FACE ( 'NONE', ( #2377 ), #21748, .T. ) ;
#13204=B_SPLINE_CURVE_WITH_KNOTS ( 'NONE', 3,
 ( #13485, #4834, #11873, #3125, #10144, #17147, #16396, #14908, #21958, #8091, #14794, #21850, #6257, #13283, #21741, #2470 ),
 .UNSPECIFIED., .F., .F.,
 ( 4, 2, 2, 2, 2, 2, 2, 4 ),
 ( 0.000000000000000000, 0.0009078963835536053763, 0.001815792767107210753, 0.002723689150660815912, 0.003631585534214421505, 0.004539481917768027099, 0.005447378301321631824, 0.007263171068428882909 ),
 .UNSPECIFIED. ) ;
#13206=DIRECTION ( 'NONE',  ( -0.01292394549866739996, -0.005513023399721131770, -0.9999012842304692006 ) ) ;
#13209=ORIENTED_EDGE ( 'NONE', *, *, #13722, .T. ) ;
#13211=CARTESIAN_POINT ( 'NONE',  ( -38.64934902010026008, 96.64904989519661171, 84.47978658464403168 ) ) ;
#13213=VERTEX_POINT ( 'NONE', #19802 ) ;
#13226=FACE_OUTER_BOUND ( 'NONE', #11605, .T. ) ;
#13227=CARTESIAN_POINT ( 'NONE',  ( -52.87539273445160148, 109.4349703648165075, -43.48703773689284446 ) ) ;
#13236=DIRECTION ( 'NONE',  ( 0.01292394549866740169, 0.005513023399720822990, 0.9999012842304693116 ) ) ;
#13237=VERTEX_POINT ( 'NONE', #9728 ) ;
#13243=CARTESIAN_POINT ( 'NONE',  ( -10.91223172713801759, 137.6763543404365180, 122.9234154551231484 ) ) ;
#13245=ORIENTED_EDGE ( 'NONE', *, *, #11390, .F. ) ;
#13261=CARTESIAN_POINT ( 'NONE',  ( -10.75874152970787634, 105.7413430127404439, 134.7986624950468126 ) ) ;
#13262=DIRECTION ( 'NONE',  ( 0.9999164797902017066, 6.965998958219365988E-18, -0.01292414190464157356 ) ) ;
#13274=AXIS2_PLACEMENT_3D ( 'NONE', #7961, #7861, #1084 ) ;
#13283=CARTESIAN_POINT ( 'NONE',  ( 47.50856862875806286, 109.5708673988121262, -44.78527194220600904 ) ) ;
#13285=VERTEX_POINT ( 'NONE', #22425 ) ;
#13286=VERTEX_POINT ( 'NONE', #3251 ) ;
#13292=ADVANCED_FACE ( 'NONE', ( #6598 ), #13623, .T. ) ;
#13301=CARTESIAN_POINT ( 'NONE',  ( 42.56450999050053952, 94.53367724843309361, 82.88992884652135729 ) ) ;
#13309=VECTOR ( 'NONE', #6293, 1000.000000000000114 ) ;
#13312=DIRECTION ( 'NONE',  ( -0.9999164797902017066, 0.000000000000000000, 0.01292414190463832269 ) ) ;
#13329=AXIS2_PLACEMENT_3D ( 'NONE', #20327, #11268, #14960 ) ;
#13332=CARTESIAN_POINT ( 'NONE',  ( -38.50312546549035631, 96.48602976677958054, 84.62394436619374005 ) ) ;
#13339=FACE_OUTER_BOUND ( 'NONE', #21448, .T. ) ;
#13341=CARTESIAN_POINT ( 'NONE',  ( -39.99665919160808869, 170.0000000000000284, 0.5169656761856410432 ) ) ;
#13342=DIRECTION ( 'NONE',  ( 7.125109674161246868E-05, -0.9999848031710253382, 0.005512562950850155054 ) ) ;
#13346=CARTESIAN_POINT ( 'NONE',  ( -49.40977258443437137, 111.5098657627030434, -43.54327172089001152 ) ) ;
#13351=DIRECTION ( 'NONE',  ( -0.01292394549866740169, -0.005513023399721021615, -0.9999012842304692006 ) ) ;
#13353=CARTESIAN_POINT ( 'NONE',  ( -10.75931153848181054, 113.7412214381086670, 134.7545619914399992 ) ) ;
#13357=DIRECTION ( 'NONE',  ( -0.01292394549866740169, -0.005513023399721130903, -0.9999012842304692006 ) ) ;
#13358=EDGE_LOOP ( 'NONE', ( #5774, #14648, #9062 ) ) ;
#13372=ORIENTED_EDGE ( 'NONE', *, *, #6553, .T. ) ;
#13387=CARTESIAN_POINT ( 'NONE',  ( 48.58946335778052372, 189.4003865961453812, -109.4536762928195230 ) ) ;
#13394=EDGE_LOOP ( 'NONE', ( #3566, #7889, #6998, #2040, #11659, #21957, #13851, #21249, #21619, #7157, #18181, #5395, #5910, #8198, #15658, #684, #15802, #6230, #7583, #17428, #21772, #8913 ) ) ;
#13396=DIRECTION ( 'NONE',  ( 0.01292394549866740169, 0.005513023399720822990, 0.9999012842304693116 ) ) ;
#13403=CARTESIAN_POINT ( 'NONE',  ( 41.32205096979155456, 107.3883277703369288, 70.91984598015065444 ) ) ;
#13406=CARTESIAN_POINT ( 'NONE',  ( -49.09819033004664846, 107.9573722685052388, 70.09443008244173257 ) ) ;
#13415=CARTESIAN_POINT ( 'NONE',  ( 49.99582398951007889, 170.0000000000000284, -0.6462070952321007367 ) ) ;
#13429=DIRECTION ( 'NONE',  ( 0.000000000000000000, -0.005512562964840580192, -0.9999848057093461140 ) ) ;
#13432=ORIENTED_EDGE ( 'NONE', *, *, #15533, .T. ) ;
#13436=CARTESIAN_POINT ( 'NONE',  ( -37.43179216281937016, 95.93806238594169145, 85.10200020414913524 ) ) ;
#13452=EDGE_LOOP ( 'NONE', ( #20260, #3851 ) ) ;
#13453=CARTESIAN_POINT ( 'NONE',  ( -52.31042862874694777, 111.8905520295979983, -46.77079012771374522 ) ) ;
#13454=ORIENTED_EDGE ( 'NONE', *, *, #17504, .F. ) ;
#13455=PLANE ( 'NONE',  #1505 ) ;
#13456=CARTESIAN_POINT ( 'NONE',  ( -10.95260071218788767, 105.6586476617446380, 119.8001432315898001 ) ) ;
#13463=DIRECTION ( 'NONE',  ( -0.01292394549866695240, -0.005513023399725255208, -0.9999012842304693116 ) ) ;
#13465=CARTESIAN_POINT ( 'NONE',  ( -42.56628114047011735, 94.99786382055523859, -43.54068532293076288 ) ) ;
#13468=DIRECTION ( 'NONE',  ( -0.01292394549866739996, -0.005513023399721131770, -0.9999012842304692006 ) ) ;
#13473=CARTESIAN_POINT ( 'NONE',  ( 47.42620204064805023, 94.99786382055523859, -44.70385809434849733 ) ) ;
#13485=CARTESIAN_POINT ( 'NONE',  ( 51.42455095033975709, 113.4816418249608034, -44.85744920025983618 ) ) ;
#13488=EDGE_CURVE ( 'NONE', #22420, #8988, #19920, .T. ) ;
#13501=ORIENTED_EDGE ( 'NONE', *, *, #11205, .T. ) ;
#13504=CARTESIAN_POINT ( 'NONE',  ( -51.19750717848778265, 189.4876967392748384, -92.32575444861939218 ) ) ;
#13506=EDGE_CURVE ( 'NONE', #7858, #16531, #17379, .T. ) ;
#13507=ORIENTED_EDGE ( 'NONE', *, *, #12756, .F. ) ;
#13508=CARTESIAN_POINT ( 'NONE',  ( -49.19269645916414646, 107.6774848903028072, 70.52757125197122434 ) ) ;
#13509=CARTESIAN_POINT ( 'NONE',  ( 42.75298547076369715, 108.3652131041115467, 57.98564716923558393 ) ) ;
#13511=DIRECTION ( 'NONE',  ( -0.9999164797902015955, -6.965998958219364448E-18, 0.01292414190464157182 ) ) ;
#13514=DIRECTION ( 'NONE',  ( -0.01292394549866695240, -0.005513023399718316314, -0.9999012842304693116 ) ) ;
#13523=LINE ( 'NONE', #3395, #14727 ) ;
#13525=ORIENTED_EDGE ( 'NONE', *, *, #20579, .F. ) ;
#13527=VECTOR ( 'NONE', #10865, 1000.000000000000000 ) ;
#13533=DIRECTION ( 'NONE',  ( 0.01292394549866737741, 0.005513023399721125699, 0.9999012842304693116 ) ) ;
#13546=LINE ( 'NONE', #8459, #19457 ) ;
#13548=AXIS2_PLACEMENT_3D ( 'NONE', #2533, #14852, #934 ) ;
#13552=PRODUCT_CONTEXT ( 'NONE', #21842, 'mechanical' ) ;
#13554=VERTEX_POINT ( 'NONE', #18099 ) ;
#13557=LINE ( 'NONE', #3192, #17701 ) ;
#13560=CARTESIAN_POINT ( 'NONE',  ( -45.67439959886510081, 164.8106407359766763, -51.88621947793163258 ) ) ;
#13565=ORIENTED_EDGE ( 'NONE', *, *, #19607, .T. ) ;
#13575=VECTOR ( 'NONE', #8799, 1000.000000000000114 ) ;
#13580=ADVANCED_FACE ( 'NONE', ( #8296 ), #1973, .F. ) ;
#13585=VERTEX_POINT ( 'NONE', #1420 ) ;
#13586=AXIS2_PLACEMENT_3D ( 'NONE', #11646, #8073, #20465 ) ;
#13597=ORIENTED_EDGE ( 'NONE', *, *, #1984, .F. ) ;
#13604=EDGE_CURVE ( 'NONE', #3576, #20464, #22396, .T. ) ;
#13609=VECTOR ( 'NONE', #15621, 999.9999999999998863 ) ;
#13616=CARTESIAN_POINT ( 'NONE',  ( -18.97922986118555500, 97.26594046717956132, 79.10430693329942642 ) ) ;
#13618=AXIS2_PLACEMENT_3D ( 'NONE', #1246, #3505, #8234 ) ;
#13620=DIRECTION ( 'NONE',  ( 0.01246513159389405628, 0.2641402835564741203, 0.9644037178988125181 ) ) ;
#13623=CYLINDRICAL_SURFACE ( 'NONE', #11524, 110.5324305509042233 ) ;
#13625=PLANE ( 'NONE',  #15918 ) ;
#13638=EDGE_LOOP ( 'NONE', ( #11978, #9408 ) ) ;
#13639=CARTESIAN_POINT ( 'NONE',  ( -38.72625626464041915, 94.79963607512176793, 84.18062813568484160 ) ) ;
#13646=CIRCLE ( 'NONE', #13274, 2.000000000000005329 ) ;
#13649=DIRECTION ( 'NONE',  ( -0.9999164797902015955, -6.965998958219364448E-18, 0.01292414190464157182 ) ) ;
#13653=CIRCLE ( 'NONE', #12556, 8.000000000000007105 ) ;
#13656=EDGE_CURVE ( 'NONE', #1745, #22420, #13204, .T. ) ;
#13659=DIRECTION ( 'NONE',  ( 0.9999164797902015955, 6.965998958219364448E-18, -0.01292414190464157182 ) ) ;
#13676=VERTEX_POINT ( 'NONE', #6033 ) ;
#13678=DIRECTION ( 'NONE',  ( -0.9999164797902015955, -6.965998958219364448E-18, 0.01292414190464157182 ) ) ;
#13681=VECTOR ( 'NONE', #8270, 1000.000000000000114 ) ;
#13684=CARTESIAN_POINT ( 'NONE',  ( -41.99321460073838352, 124.0006990541328804, 0.7963918557340313731 ) ) ;
#13687=CARTESIAN_POINT ( 'NONE',  ( 51.31288912873903740, 109.9913629100859254, -44.83676205748413679 ) ) ;
#13694=CIRCLE ( 'NONE', #18458, 7.499999999999991118 ) ;
#13708=DIRECTION ( 'NONE',  ( -0.9999164797902015955, -6.965998958219364448E-18, 0.01292414190464157182 ) ) ;
#13719=CARTESIAN_POINT ( 'NONE',  ( 28.96536656690224021, 99.74539563421257071, 74.50764472524521409 ) ) ;
#13720=DIRECTION ( 'NONE',  ( 0.9999164797902014845, 0.000000000000000000, -0.01292414190465219874 ) ) ;
#13722=EDGE_CURVE ( 'NONE', #15636, #2773, #12644, .T. ) ;
#13728=VERTEX_POINT ( 'NONE', #19381 ) ;
#13732=CARTESIAN_POINT ( 'NONE',  ( -24.71812196488931690, 189.4003865961453528, -108.5061595206230720 ) ) ;
#13746=CARTESIAN_POINT ( 'NONE',  ( -52.03388546434464246, 189.5999951618935597, -71.94389034825996987 ) ) ;
#13760=ORIENTED_EDGE ( 'NONE', *, *, #9779, .T. ) ;
#13776=CARTESIAN_POINT ( 'NONE',  ( 44.31784132852413194, 168.2105890667581605, -53.06813496338226344 ) ) ;
#13785=CARTESIAN_POINT ( 'NONE',  ( -48.67164386273223187, 109.5652376256254854, -43.54209035921780213 ) ) ;
#13786=CARTESIAN_POINT ( 'NONE',  ( -65.59152507611121052, 113.4706157781613598, -45.34512716587771308 ) ) ;
#13795=CARTESIAN_POINT ( 'NONE',  ( 47.76182451837959064, 110.4323045661290337, -44.79329492277620517 ) ) ;
#13797=CARTESIAN_POINT ( 'NONE',  ( 41.22194066120597000, 125.3750519639578727, 249.0299023193002768 ) ) ;
#13801=ORIENTED_EDGE ( 'NONE', *, *, #20006, .T. ) ;
#13805=CARTESIAN_POINT ( 'NONE',  ( 49.23668000689734470, 95.70300605291201634, -45.90578145146270117 ) ) ;
#13806=FACE_OUTER_BOUND ( 'NONE', #14341, .T. ) ;
#13813=EDGE_LOOP ( 'NONE', ( #14537, #6693, #4633, #11977 ) ) ;
#13814=EDGE_LOOP ( 'NONE', ( #2032, #7822, #5738, #611 ) ) ;
#13820=DIRECTION ( 'NONE',  ( -0.01292394549866740690, -0.005513023399721241925, -0.9999012842304693116 ) ) ;
#13825=LINE ( 'NONE', #16022, #20678 ) ;
#13832=DIRECTION ( 'NONE',  ( -0.01292394549866740169, -0.005513023399721021615, -0.9999012842304692006 ) ) ;
#13838=DIRECTION ( 'NONE',  ( 0.9999164797902015955, 6.965998958219364448E-18, -0.01292414190464157182 ) ) ;
#13839=EDGE_CURVE ( 'NONE', #13165, #20787, #10415, .T. ) ;
#13845=CARTESIAN_POINT ( 'NONE',  ( 43.19632491693555210, 119.7615706795621691, 247.0351358235509167 ) ) ;
#13847=CARTESIAN_POINT ( 'NONE',  ( -52.93127853433226448, 189.6011917897851333, -71.71522176735570042 ) ) ;
#13851=ORIENTED_EDGE ( 'NONE', *, *, #15823, .T. ) ;
#13869=CARTESIAN_POINT ( 'NONE',  ( 48.79414080053240355, 189.4876967392748384, -93.61816863908353525 ) ) ;
#13881=DIRECTION ( 'NONE',  ( 0.9999164797902015955, 6.965998958219364448E-18, -0.01292414190464157182 ) ) ;
#13890=ORIENTED_EDGE ( 'NONE', *, *, #16286, .T. ) ;
#13893=SPHERICAL_SURFACE ( 'NONE', #16560, 2.000000000000000000 ) ;
#13897=CARTESIAN_POINT ( 'NONE',  ( -51.97046013708073531, 113.4377915441418452, -43.52080401654976072 ) ) ;
#13898=ORIENTED_EDGE ( 'NONE', *, *, #12847, .T. ) ;
#13899=CARTESIAN_POINT ( 'NONE',  ( 50.82209241344880724, 113.4364193371377638, -44.84941295302596131 ) ) ;
#13904=VERTEX_POINT ( 'NONE', #12747 ) ;
#13913=VERTEX_POINT ( 'NONE', #20908 ) ;
#13914=CARTESIAN_POINT ( 'NONE',  ( -66.19625437534079992, 189.4876967392748384, -92.13189232004975793 ) ) ;
#13925=AXIS2_PLACEMENT_3D ( 'NONE', #15256, #3255, #6720 ) ;
#13949=CARTESIAN_POINT ( 'NONE',  ( -65.56790548363530036, 144.7550503794368524, -43.51772385068294113 ) ) ;
#13950=CARTESIAN_POINT ( 'NONE',  ( 49.99582398951007889, 170.0000000000000284, -0.6462070952321007367 ) ) ;
#13956=CARTESIAN_POINT ( 'NONE',  ( -51.42204038937180144, 189.5972346270502271, -72.45256254838918153 ) ) ;
#13971=VECTOR ( 'NONE', #3950, 1000.000000000000114 ) ;
#13985=DIRECTION ( 'NONE',  ( 0.01292394549866738261, 0.005513023399722618428, 0.9999012842304692006 ) ) ;
#13994=AXIS2_PLACEMENT_3D ( 'NONE', #2810, #9713, #16624 ) ;
#14002=DIRECTION ( 'NONE',  ( -7.125109674243555432E-05, 0.9999848031710253382, -0.005512562950850175003 ) ) ;
#14013=EDGE_CURVE ( 'NONE', #1999, #7226, #9693, .T. ) ;
#14023=CARTESIAN_POINT ( 'NONE',  ( 49.79948073228538874, 109.1696245789948847, -44.81267020896142839 ) ) ;
#14024=CIRCLE ( 'NONE', #4097, 7.499999999999991118 ) ;
#14029=DIRECTION ( 'NONE',  ( -0.01292394549866737914, -0.005513023399721009472, -0.9999012842304692006 ) ) ;
#14032=ORIENTED_EDGE ( 'NONE', *, *, #10021, .T. ) ;
#14034=FACE_BOUND ( 'NONE', #4289, .T. ) ;
#14036=CIRCLE ( 'NONE', #4832, 110.5000000000000142 ) ;
#14044=AXIS2_PLACEMENT_3D ( 'NONE', #13117, #16576, #21911 ) ;
#14046=EDGE_CURVE ( 'NONE', #4037, #14965, #21933, .T. ) ;
#14049=DIRECTION ( 'NONE',  ( -7.125109674243555432E-05, 0.9999848031710253382, -0.005512562950850175003 ) ) ;
#14056=VERTEX_POINT ( 'NONE', #6227 ) ;
#14071=AXIS2_PLACEMENT_3D ( 'NONE', #7420, #14337, #19252 ) ;
#14079=DIRECTION ( 'NONE',  ( 7.125109674161246868E-05, -0.9999848031710252272, 0.005512562950850154186 ) ) ;
#14107=DIRECTION ( 'NONE',  ( 0.9999164797902017066, 6.965998958219365988E-18, -0.01292414190464157356 ) ) ;
#14114=CARTESIAN_POINT ( 'NONE',  ( 52.39275651943277268, 106.8510597072923218, 70.21618947625844953 ) ) ;
#14120=TOROIDAL_SURFACE ( 'NONE', #21439, 77.00000000000002842, 2.000000000000000000 ) ;
#14129=EDGE_CURVE ( 'NONE', #19370, #14056, #7, .T. ) ;
#14133=ADVANCED_FACE ( 'NONE', ( #12320 ), #15215, .F. ) ;
#14143=CARTESIAN_POINT ( 'NONE',  ( -50.61043681403349837, 112.8347543081579403, -43.53505773252739175 ) ) ;
#14152=ADVANCED_FACE ( 'NONE', ( #13339 ), #22133, .T. ) ;
#14159=PLANE ( 'NONE',  #4702 ) ;
#14163=ORIENTED_EDGE ( 'NONE', *, *, #21880, .F. ) ;
#14169=DIRECTION ( 'NONE',  ( -0.9999164797902015955, -6.965998958219364448E-18, 0.01292414190464157182 ) ) ;
#14172=DIRECTION ( 'NONE',  ( -0.01292394549866740169, -0.005513023399721277487, -0.9999012842304693116 ) ) ;
#14174=ORIENTED_EDGE ( 'NONE', *, *, #15743, .T. ) ;
#14176=CARTESIAN_POINT ( 'NONE',  ( -45.67464185259402853, 168.2105890667581605, -51.90496219196452188 ) ) ;
#14180=LINE ( 'NONE', #17395, #20930 ) ;
#14181=EDGE_LOOP ( 'NONE', ( #4093, #15086, #18273, #17409, #6300 ) ) ;
#14182=DIRECTION ( 'NONE',  ( -0.01292394549867042185, -0.005513023399725255208, -0.9999012842304693116 ) ) ;
#14183=FILL_AREA_STYLE_COLOUR ( '', #17813 ) ;
#14199=DIRECTION ( 'NONE',  ( -0.009188991635466048358, 0.7031977391749438810, -0.7109349492407661675 ) ) ;
#14208=LINE ( 'NONE', #12248, #7723 ) ;
#14211=DIRECTION ( 'NONE',  ( -0.01246513159389404414, -0.2641402835564772844, -0.9644037178988117409 ) ) ;
#14227=AXIS2_PLACEMENT_3D ( 'NONE', #3258, #10284, #13206 ) ;
#14228=CARTESIAN_POINT ( 'NONE',  ( 51.30310378538536042, 107.3244244979011057, 69.70064189502821250 ) ) ;
#14233=EDGE_LOOP ( 'NONE', ( #229, #13432, #14295, #9335 ) ) ;
#14246=CARTESIAN_POINT ( 'NONE',  ( 51.38234815825343560, 111.9218655255082382, -48.12259961501337102 ) ) ;
#14247=ORIENTED_EDGE ( 'NONE', *, *, #20397, .F. ) ;
#14249=ORIENTED_EDGE ( 'NONE', *, *, #18616, .T. ) ;
#14251=CARTESIAN_POINT ( 'NONE',  ( -52.26459910193298697, 113.4816418249607750, -43.51724397679114276 ) ) ;
#14259=FACE_OUTER_BOUND ( 'NONE', #3119, .T. ) ;
#14265=CARTESIAN_POINT ( 'NONE',  ( 42.91324393340197219, 106.8060942374655156, 70.38454212103849272 ) ) ;
#14268=ADVANCED_FACE ( 'NONE', ( #19790 ), #9244, .T. ) ;
#14285=VERTEX_POINT ( 'NONE', #10661 ) ;
#14295=ORIENTED_EDGE ( 'NONE', *, *, #3526, .T. ) ;
#14305=EDGE_CURVE ( 'NONE', #19636, #2746, #21932, .T. ) ;
#14306=CARTESIAN_POINT ( 'NONE',  ( 49.42284594772163331, 139.7551263635817236, -44.97643735496247785 ) ) ;
#14309=CARTESIAN_POINT ( 'NONE',  ( 39.46073478354046671, 96.01222662467367286, -42.85086330523944298 ) ) ;
#14313=CARTESIAN_POINT ( 'NONE',  ( -38.48616300399660162, 94.99421645999460395, 83.38067543124275005 ) ) ;
#14314=EDGE_CURVE ( 'NONE', #883, #15636, #8958, .T. ) ;
#14322=CIRCLE ( 'NONE', #20511, 3.999999999999999556 ) ;
#14328=LINE ( 'NONE', #3852, #13527 ) ;
#14333=AXIS2_PLACEMENT_3D ( 'NONE', #18789, #1453, #22538 ) ;
#14335=CARTESIAN_POINT ( 'NONE',  ( -64.99457118636313169, 170.0000000000000284, 0.8400692238016805868 ) ) ;
#14337=DIRECTION ( 'NONE',  ( -7.125109674161231961E-05, 0.9999848031710252272, -0.005512562950850142043 ) ) ;
#14341=EDGE_LOOP ( 'NONE', ( #18959, #1353, #17666, #1145, #344 ) ) ;
#14355=SPHERICAL_SURFACE ( 'NONE', #10273, 2.000000000000000000 ) ;
#14370=DIRECTION ( 'NONE',  ( 0.9999164797902015955, 6.965998958219364448E-18, -0.01292414190464157182 ) ) ;
#14371=ORIENTED_EDGE ( 'NONE', *, *, #21105, .T. ) ;
#14374=VECTOR ( 'NONE', #7625, 1000.000000000000000 ) ;
#14380=DIRECTION ( 'NONE',  ( -0.01292394549866740169, -0.005513023399719847208, -0.9999012842304693116 ) ) ;
#14385=VERTEX_POINT ( 'NONE', #21851 ) ;
#14408=CARTESIAN_POINT ( 'NONE',  ( 49.82165995907426037, 189.5987917270899459, -73.47870018378864643 ) ) ;
#14411=CIRCLE ( 'NONE', #4462, 2.000000000000001332 ) ;
#14414=CARTESIAN_POINT ( 'NONE',  ( 64.42259306105445660, 139.7551263635816952, -45.17031240767400391 ) ) ;
#14417=CARTESIAN_POINT ( 'NONE',  ( 41.20362701579343678, 107.2712125007551691, 92.86385812504968840 ) ) ;
#14420=CIRCLE ( 'NONE', #14785, 87.00000000000001421 ) ;
#14421=CARTESIAN_POINT ( 'NONE',  ( 41.19638261157623305, 121.2962013336460814, 247.0525242307099347 ) ) ;
#14434=DIRECTION ( 'NONE',  ( 7.125109674161446091E-05, -0.9999848031710252272, 0.005512562950850307709 ) ) ;
#14445=CIRCLE ( 'NONE', #15547, 112.5000000000000142 ) ;
#14449=ADVANCED_FACE ( 'NONE', ( #16397 ), #15311, .F. ) ;
#14453=EDGE_CURVE ( 'NONE', #5372, #22420, #10052, .T. ) ;
#14455=CARTESIAN_POINT ( 'NONE',  ( 23.17824588921087781, -5.346239964818104262, -10.63114771928880309 ) ) ;
#14467=DIRECTION ( 'NONE',  ( 7.125109674161246868E-05, -0.9999848031710252272, 0.005512562950850154186 ) ) ;
#14468=CARTESIAN_POINT ( 'NONE',  ( 52.91240873130399081, 106.8060942374655156, 70.25530070199208410 ) ) ;
#14482=DIRECTION ( 'NONE',  ( -0.01292394549866739996, -0.005513023399721118760, -0.9999012842304692006 ) ) ;
#14483=EDGE_CURVE ( 'NONE', #9660, #2844, #534, .T. ) ;
#14486=VECTOR ( 'NONE', #17130, 999.9999999999998863 ) ;
#14499=CARTESIAN_POINT ( 'NONE',  ( -40.55508067841016384, 96.01222808543204223, -41.81663866985299194 ) ) ;
#14503=ADVANCED_FACE ( 'NONE', ( #22417 ), #14120, .F. ) ;
#14510=ORIENTED_EDGE ( 'NONE', *, *, #8479, .F. ) ;
#14512=DIRECTION ( 'NONE',  ( -0.9999164797902017066, -6.965998958219367529E-18, 0.01292414190464157182 ) ) ;
#14517=EDGE_LOOP ( 'NONE', ( #241, #3504, #2057, #2998 ) ) ;
#14521=CARTESIAN_POINT ( 'NONE',  ( 49.44092383899086229, 189.5967114759612286, -73.85113886024416274 ) ) ;
#14526=DIRECTION ( 'NONE',  ( -0.01292394549866695240, -0.005513023399718316314, -0.9999012842304693116 ) ) ;
#14533=VECTOR ( 'NONE', #16343, 1000.000000000000000 ) ;
#14537=ORIENTED_EDGE ( 'NONE', *, *, #4996, .F. ) ;
#14539=DIRECTION ( 'NONE',  ( 0.9999164797902015955, 6.965998958219364448E-18, -0.01292414190464157182 ) ) ;
#14554=ORIENTED_EDGE ( 'NONE', *, *, #853, .T. ) ;
#14558=DIRECTION ( 'NONE',  ( -0.01292394549866744159, -0.005513023399721009472, -0.9999012842304692006 ) ) ;
#14566=EDGE_CURVE ( 'NONE', #22043, #2491, #6490, .T. ) ;
#14579=ORIENTED_EDGE ( 'NONE', *, *, #10497, .F. ) ;
#14589=ADVANCED_FACE ( 'NONE', ( #9215, #12570 ), #17871, .F. ) ;
#14594=CARTESIAN_POINT ( 'NONE',  ( -10.85795115604361349, 137.6995090387153482, 127.1230008488911096 ) ) ;
#14595=CARTESIAN_POINT ( 'NONE',  ( 49.39754356754257714, 108.7350236001487502, -46.93403478043238408 ) ) ;
#14600=DIRECTION ( 'NONE',  ( 0.009188991635466050092, -0.7031977391749439921, 0.7109349492407662785 ) ) ;
#14609=CIRCLE ( 'NONE', #6861, 1.999999999999998446 ) ;
#14615=VERTEX_POINT ( 'NONE', #3706 ) ;
#14621=LINE ( 'NONE', #21576, #3401 ) ;
#14629=ORIENTED_EDGE ( 'NONE', *, *, #9209, .T. ) ;
#14635=EDGE_LOOP ( 'NONE', ( #20281, #22184, #1826, #19140 ) ) ;
#14648=ORIENTED_EDGE ( 'NONE', *, *, #16007, .T. ) ;
#14650=CARTESIAN_POINT ( 'NONE',  ( 40.75315251118328774, 108.3652131041115467, 58.01149545304486566 ) ) ;
#14651=CARTESIAN_POINT ( 'NONE',  ( 40.73863394693862006, 95.06543039568907716, -44.50011052238011189 ) ) ;
#14653=CIRCLE ( 'NONE', #3615, 87.00000000000001421 ) ;
#14665=CARTESIAN_POINT ( 'NONE',  ( -49.09967157776827662, 108.0238286078847523, 69.97982874036236467 ) ) ;
#14671=CARTESIAN_POINT ( 'NONE',  ( -26.94222022802838268, 95.51270090492251086, 82.01937116434973518 ) ) ;
#14675=CARTESIAN_POINT ( 'NONE',  ( 49.99582398951009310, 170.0000000000008242, -0.6462070952312342076 ) ) ;
#14676=ORIENTED_EDGE ( 'NONE', *, *, #16007, .F. ) ;
#14685=ADVANCED_FACE ( 'NONE', ( #16349 ), #21681, .T. ) ;
#14689=AXIS2_PLACEMENT_3D ( 'NONE', #13776, #1816, #14002 ) ;
#14691=DIRECTION ( 'NONE',  ( -0.9999164797902017066, -6.965998958219365988E-18, 0.01292414190464157356 ) ) ;
#14699=EDGE_CURVE ( 'NONE', #1745, #1664, #1303, .T. ) ;
#14704=ORIENTED_EDGE ( 'NONE', *, *, #21966, .T. ) ;
#14707=CARTESIAN_POINT ( 'NONE',  ( -35.41995824635180412, 106.0982379271226677, 199.8585325857761177 ) ) ;
#14716=ORIENTED_EDGE ( 'NONE', *, *, #2520, .T. ) ;
#14717=DIRECTION ( 'NONE',  ( -0.01292394549866737220, -0.005513023399721000799, -0.9999012842304692006 ) ) ;
#14718=CARTESIAN_POINT ( 'NONE',  ( 51.42455095033975709, 113.4816418249608034, -44.85744920025983618 ) ) ;
#14727=VECTOR ( 'NONE', #15266, 1000.000000000000000 ) ;
#14736=TOROIDAL_SURFACE ( 'NONE', #785, 110.5000000000000000, 2.000000000000000000 ) ;
#14737=CARTESIAN_POINT ( 'NONE',  ( -51.81996628516554182, 111.6265379432125684, -46.67980995128849031 ) ) ;
#14739=DIRECTION ( 'NONE',  ( 0.01292394549866695240, 0.005513023399725255208, 0.9999012842304693116 ) ) ;
#14747=ADVANCED_FACE ( 'NONE', ( #16892 ), #9871, .F. ) ;
#14749=AXIS2_PLACEMENT_3D ( 'NONE', #18237, #16947, #20471 ) ;
#14756=CARTESIAN_POINT ( 'NONE',  ( 43.10250357860363835, 95.91520285510637223, 84.25345810160554549 ) ) ;
#14761=AXIS2_PLACEMENT_3D ( 'NONE', #20468, #15338, #11881 ) ;
#14766=AXIS2_PLACEMENT_3D ( 'NONE', #12925, #12462, #14771 ) ;
#14771=DIRECTION ( 'NONE',  ( -7.125109674243555432E-05, 0.9999848031710253382, -0.005512562950850175003 ) ) ;
#14777=EDGE_CURVE ( 'NONE', #9718, #8189, #18168, .T. ) ;
#14780=VECTOR ( 'NONE', #4922, 1000.000000000000000 ) ;
#14785=AXIS2_PLACEMENT_3D ( 'NONE', #11530, #22056, #17049 ) ;
#14789=AXIS2_PLACEMENT_3D ( 'NONE', #15299, #8593, #18933 ) ;
#14794=CARTESIAN_POINT ( 'NONE',  ( 48.11994755510385602, 111.2501766408243498, -44.80243313535611804 ) ) ;
#14801=DIRECTION ( 'NONE',  ( -0.9999164797902015955, -6.965998958219364448E-18, 0.01292414190464157182 ) ) ;
#14807=CARTESIAN_POINT ( 'NONE',  ( -40.95677474166659238, 106.8061942917681790, 71.46866982798410106 ) ) ;
#14812=ORIENTED_EDGE ( 'NONE', *, *, #21972, .T. ) ;
#14825=AXIS2_PLACEMENT_3D ( 'NONE', #2765, #1163, #6540 ) ;
#14827=ORIENTED_EDGE ( 'NONE', *, *, #18596, .T. ) ;
#14831=ORIENTED_EDGE ( 'NONE', *, *, #10058, .T. ) ;
#14838=DIRECTION ( 'NONE',  ( 0.01292394549866740169, 0.005513023399719847208, 0.9999012842304693116 ) ) ;
#14846=EDGE_CURVE ( 'NONE', #17586, #8873, #15058, .T. ) ;
#14851=VECTOR ( 'NONE', #5277, 999.9999999999998863 ) ;
#14852=DIRECTION ( 'NONE',  ( 0.9999164797902017066, 6.965998958219365988E-18, -0.01292414190464157356 ) ) ;
#14853=CARTESIAN_POINT ( 'NONE',  ( -51.02393100784042446, 110.5294973102531770, -46.28750279846238413 ) ) ;
#14864=DIRECTION ( 'NONE',  ( 7.125109674161246868E-05, -0.9999848031710252272, 0.005512562950850154186 ) ) ;
#14866=VECTOR ( 'NONE', #15755, 1000.000000000000227 ) ;
#14870=CARTESIAN_POINT ( 'NONE',  ( 39.99665919160806027, 170.0000000000000284, -0.5169656761856848970 ) ) ;
#14873=CARTESIAN_POINT ( 'NONE',  ( -51.47772934420782320, 111.2940323025706846, -46.56188176222278940 ) ) ;
#14886=CARTESIAN_POINT ( 'NONE',  ( -37.08415557685306396, 105.5218503240047454, 92.65813065591969178 ) ) ;
#14887=CARTESIAN_POINT ( 'NONE',  ( -52.56676294784124792, 113.4816418249608034, -43.51333844217711544 ) ) ;
#14889=CARTESIAN_POINT ( 'NONE',  ( 47.39940051867662874, 108.3707227317548529, -46.77744129239903259 ) ) ;
#14893=ORIENTED_EDGE ( 'NONE', *, *, #853, .F. ) ;
#14899=FACE_OUTER_BOUND ( 'NONE', #3029, .T. ) ;
#14901=ORIENTED_EDGE ( 'NONE', *, *, #7695, .F. ) ;
#14903=DIRECTION ( 'NONE',  ( 0.009188991635466048358, -0.7031977391749438810, 0.7109349492407661675 ) ) ;
#14908=CARTESIAN_POINT ( 'NONE',  ( 48.79856628852573408, 112.2275063344195303, -44.81659300615380204 ) ) ;
#14911=ORIENTED_EDGE ( 'NONE', *, *, #10520, .T. ) ;
#14923=CARTESIAN_POINT ( 'NONE',  ( -39.75561905526965489, 107.1788419875363303, 71.78347329497708529 ) ) ;
#14926=EDGE_CURVE ( 'NONE', #2396, #20375, #3431, .T. ) ;
#14939=VERTEX_POINT ( 'NONE', #17693 ) ;
#14940=ORIENTED_EDGE ( 'NONE', *, *, #12756, .T. ) ;
#14946=DIRECTION ( 'NONE',  ( -0.9999164797902015955, -6.965998958219364448E-18, 0.01292414190464157182 ) ) ;
#14951=EDGE_LOOP ( 'NONE', ( #115, #16594, #1334, #18316 ) ) ;
#14957=CARTESIAN_POINT ( 'NONE',  ( -52.26439264322070954, 113.4816418191338414, -43.51724664528359909 ) ) ;
#14960=DIRECTION ( 'NONE',  ( 0.01292394549866738261, 0.005513023399722618428, 0.9999012842304692006 ) ) ;
#14965=VERTEX_POINT ( 'NONE', #3770 ) ;
#14970=EDGE_CURVE ( 'NONE', #8421, #7828, #1599, .T. ) ;
#14972=DIRECTION ( 'NONE',  ( -0.009088227368120585167, -0.7109943316365089361, -0.7031390079522393810 ) ) ;
#14974=ORIENTED_EDGE ( 'NONE', *, *, #14046, .F. ) ;
#14984=EDGE_CURVE ( 'NONE', #16331, #16712, #12295, .T. ) ;
#14989=CARTESIAN_POINT ( 'NONE',  ( -36.86384537466776834, 93.14505924924313263, 85.22952222962540247 ) ) ;
#15001=DIRECTION ( 'NONE',  ( -0.9999164797902017066, -6.965998958219365988E-18, 0.01292414190464157356 ) ) ;
#15010=VERTEX_POINT ( 'NONE', #18031 ) ;
#15020=ORIENTED_EDGE ( 'NONE', *, *, #15487, .T. ) ;
#15029=AXIS2_PLACEMENT_3D ( 'NONE', #7460, #5833, #1956 ) ;
#15035=EDGE_LOOP ( 'NONE', ( #9824, #11507, #8984, #2555 ) ) ;
#15058=LINE ( 'NONE', #22017, #18423 ) ;
#15059=EDGE_CURVE ( 'NONE', #9820, #22544, #12947, .T. ) ;
#15060=CIRCLE ( 'NONE', #376, 2.000000000000005329 ) ;
#15070=CARTESIAN_POINT ( 'NONE',  ( 14.14224087380716455, 105.6999953372425409, 126.9762993157022777 ) ) ;
#15076=PLANE ( 'NONE',  #11741 ) ;
#15082=FACE_OUTER_BOUND ( 'NONE', #7774, .T. ) ;
#15086=ORIENTED_EDGE ( 'NONE', *, *, #20473, .T. ) ;
#15088=DIRECTION ( 'NONE',  ( 0.01292394549866743812, 0.005513023399720639109, 0.9999012842304693116 ) ) ;
#15090=ORIENTED_EDGE ( 'NONE', *, *, #4704, .T. ) ;
#15118=AXIS2_PLACEMENT_3D ( 'NONE', #18633, #11637, #2893 ) ;
#15119=CARTESIAN_POINT ( 'NONE',  ( -49.99582398951010731, 170.0000000000000284, 0.6462070952320568828 ) ) ;
#15134=CARTESIAN_POINT ( 'NONE',  ( -49.28939966538133888, 107.5356485694709789, 70.72646220445905385 ) ) ;
#15141=DIRECTION ( 'NONE',  ( -0.01292394549866737914, -0.005513023399721009472, -0.9999012842304692006 ) ) ;
#15142=DIRECTION ( 'NONE',  ( 0.9999164797902017066, 6.965998958219367529E-18, -0.01292414190464157182 ) ) ;
#15162=EDGE_CURVE ( 'NONE', #444, #21389, #1463, .T. ) ;
#15177=VECTOR ( 'NONE', #6414, 1000.000000000000114 ) ;
#15185=AXIS2_PLACEMENT_3D ( 'NONE', #13415, #15142, #15586 ) ;
#15188=ORIENTED_EDGE ( 'NONE', *, *, #19618, .T. ) ;
#15191=ORIENTED_EDGE ( 'NONE', *, *, #9701, .F. ) ;
#15195=FACE_OUTER_BOUND ( 'NONE', #16150, .T. ) ;
#15196=DIRECTION ( 'NONE',  ( 0.01292394549866739996, 0.005513023399721564584, 0.9999012842304692006 ) ) ;
#15211=DIRECTION ( 'NONE',  ( 0.9999164797902015955, 6.965998958219364448E-18, -0.01292414190464157182 ) ) ;
#15215=TOROIDAL_SURFACE ( 'NONE', #4906, 93.00000000000000000, 2.000000000000000000 ) ;
#15225=AXIS2_PLACEMENT_3D ( 'NONE', #16221, #11015, #14717 ) ;
#15226=CARTESIAN_POINT ( 'NONE',  ( 64.42346518761236496, 113.4816418249608034, -45.02546304502017449 ) ) ;
#15228=CARTESIAN_POINT ( 'NONE',  ( -52.67340511173117079, 189.4880640929450237, -92.24003979316276514 ) ) ;
#15240=DIRECTION ( 'NONE',  ( 0.01292394549866740169, 0.005513023399720822990, 0.9999012842304693116 ) ) ;
#15247=AXIS2_PLACEMENT_3D ( 'NONE', #1277, #10211, #8264 ) ;
#15256=CARTESIAN_POINT ( 'NONE',  ( -46.77031037318527495, 119.7725967263615985, 250.1981111634296155 ) ) ;
#15259=PLANE ( 'NONE',  #15185 ) ;
#15264=EDGE_CURVE ( 'NONE', #18464, #18018, #8000, .T. ) ;
#15266=DIRECTION ( 'NONE',  ( -0.9999164797902015955, -6.965998958219364448E-18, 0.01292414190464157182 ) ) ;
#15268=ORIENTED_EDGE ( 'NONE', *, *, #8933, .F. ) ;
#15274=ADVANCED_FACE ( 'NONE', ( #6513 ), #15378, .T. ) ;
#15281=ORIENTED_EDGE ( 'NONE', *, *, #9343, .F. ) ;
#15282=DIRECTION ( 'NONE',  ( -0.01292394549866744159, -0.005513023399721009472, -0.9999012842304692006 ) ) ;
#15285=CARTESIAN_POINT ( 'NONE',  ( 19.42556530730579567, 136.7551719540686008, -44.57217540897067920 ) ) ;
#15299=CARTESIAN_POINT ( 'NONE',  ( -64.99457118636313169, 170.0000000000000284, 0.8400692238016805868 ) ) ;
#15310=FACE_OUTER_BOUND ( 'NONE', #10818, .T. ) ;
#15311=( BOUNDED_SURFACE ( )  B_SPLINE_SURFACE ( 3, 3, ( 
 ( #14671, #21624, #12949, #18221 ),
 ( #7755, #6034, #20032, #13732 ),
 ( #13616, #4858, #16958, #20599 ),
 ( #15464, #18987, #11776, #8416 ) ),
 .UNSPECIFIED., .F., .F., .T. ) 
 B_SPLINE_SURFACE_WITH_KNOTS ( ( 4, 4 ),
 ( 4, 4 ),
 ( 0.000000000000000000, 1.000000000000000000 ),
 ( 0.000000000000000000, 1.000000000000000000 ),
 .UNSPECIFIED. ) 
 GEOMETRIC_REPRESENTATION_ITEM ( )  RATIONAL_B_SPLINE_SURFACE ( (
 ( 1.000000000000000000, 0.5185431720251972854, 0.5185431720251972854, 1.000000000000000000),
 ( 0.8047378541243649375, 0.4172913195263986963, 0.4172913195263986963, 0.8047378541243649375),
 ( 0.8047378541243649375, 0.4172913195263986963, 0.4172913195263986963, 0.8047378541243649375),
 ( 1.000000000000000000, 0.5185431720251972854, 0.5185431720251972854, 1.000000000000000000) ) ) 
 REPRESENTATION_ITEM ( '' )  SURFACE ( )  );
#15316=DIRECTION ( 'NONE',  ( 0.01292394549866737741, 0.005513023399721125699, 0.9999012842304693116 ) ) ;
#15320=CYLINDRICAL_SURFACE ( 'NONE', #4101, 95.00000000000001421 ) ;
#15321=ORIENTED_EDGE ( 'NONE', *, *, #7734, .F. ) ;
#15324=ORIENTED_EDGE ( 'NONE', *, *, #14483, .T. ) ;
#15335=CYLINDRICAL_SURFACE ( 'NONE', #9906, 2.000000000000001332 ) ;
#15338=DIRECTION ( 'NONE',  ( 7.125109674161246868E-05, -0.9999848031710252272, 0.005512562950850154186 ) ) ;
#15343=CARTESIAN_POINT ( 'NONE',  ( 26.69469236638542853, 189.4444907833431273, -101.1701348970736518 ) ) ;
#15346=ORIENTED_EDGE ( 'NONE', *, *, #11528, .T. ) ;
#15361=FACE_OUTER_BOUND ( 'NONE', #14233, .T. ) ;
#15363=CARTESIAN_POINT ( 'NONE',  ( 41.99976970163857715, 124.0006990541328804, -0.2892360642558610695 ) ) ;
#15368=CARTESIAN_POINT ( 'NONE',  ( -40.43344728539147326, 106.8827357009993051, 71.53004524236550310 ) ) ;
#15371=CARTESIAN_POINT ( 'NONE',  ( -39.02517588049546049, 94.68893737706953573, 84.08474196546899293 ) ) ;
#15377=VECTOR ( 'NONE', #12237, 999.9999999999998863 ) ;
#15378=CYLINDRICAL_SURFACE ( 'NONE', #16981, 110.5324305509042233 ) ;
#15383=ORIENTED_EDGE ( 'NONE', *, *, #15059, .T. ) ;
#15384=LINE ( 'NONE', #1697, #8745 ) ;
#15391=VERTEX_POINT ( 'NONE', #5339 ) ;
#15396=CARTESIAN_POINT ( 'NONE',  ( 39.18815798788130422, 105.5072037373731888, 91.67997329703011644 ) ) ;
#15398=CARTESIAN_POINT ( 'NONE',  ( -34.79726985247908999, 121.2962013336460814, 248.0347590154626971 ) ) ;
#15410=CYLINDRICAL_SURFACE ( 'NONE', #21898, 3.399999999999985700 ) ;
#15411=LINE ( 'NONE', #3311, #20962 ) ;
#15416=VERTEX_POINT ( 'NONE', #19469 ) ;
#15417=CARTESIAN_POINT ( 'NONE',  ( 49.57492634055867597, 108.8066997800019351, -44.80776678329138463 ) ) ;
#15430=CYLINDRICAL_SURFACE ( 'NONE', #1889, 87.00000000000001421 ) ;
#15437=CARTESIAN_POINT ( 'NONE',  ( 64.99457118636310327, 170.0000000000000284, -0.8400692238017243296 ) ) ;
#15459=EDGE_CURVE ( 'NONE', #20375, #4427, #8101, .T. ) ;
#15464=CARTESIAN_POINT ( 'NONE',  ( -19.03062446302745414, 99.74539563421258492, 75.12800353666801811 ) ) ;
#15473=AXIS2_PLACEMENT_3D ( 'NONE', #6999, #15754, #22259 ) ;
#15477=LINE ( 'NONE', #13845, #12986 ) ;
#15480=CARTESIAN_POINT ( 'NONE',  ( -51.01306968729422664, 189.5926701885510397, -73.28584260091861324 ) ) ;
#15482=CARTESIAN_POINT ( 'NONE',  ( -10.85567112094788200, 105.6999953372425409, 127.2994028633183063 ) ) ;
#15485=FACE_OUTER_BOUND ( 'NONE', #5286, .T. ) ;
#15487=EDGE_CURVE ( 'NONE', #12735, #22296, #12714, .T. ) ;
#15491=AXIS2_PLACEMENT_3D ( 'NONE', #14421, #19327, #21380 ) ;
#15509=DIRECTION ( 'NONE',  ( 0.01292394549866695240, 0.005513023399725255208, 0.9999012842304693116 ) ) ;
#15512=CARTESIAN_POINT ( 'NONE',  ( -41.23999883161326352, 108.3652131041115467, 59.07127508922548031 ) ) ;
#15519=CARTESIAN_POINT ( 'NONE',  ( -48.56673365018540522, 108.3817487785542539, -43.53692110109250279 ) ) ;
#15521=DIRECTION ( 'NONE',  ( -0.9999164797902015955, -6.965998958219364448E-18, 0.01292414190464157182 ) ) ;
#15525=CARTESIAN_POINT ( 'NONE',  ( -48.56675504324970660, 108.6819931279166838, -43.53857624212188426 ) ) ;
#15526=EDGE_LOOP ( 'NONE', ( #12147, #3003, #13041, #3174 ) ) ;
#15533=EDGE_CURVE ( 'NONE', #21686, #5966, #4069, .T. ) ;
#15547=AXIS2_PLACEMENT_3D ( 'NONE', #1133, #13649, #13533 ) ;
#15551=DIRECTION ( 'NONE',  ( 0.01292394549866740169, 0.005513023399720822990, 0.9999012842304693116 ) ) ;
#15557=ORIENTED_EDGE ( 'NONE', *, *, #16847, .T. ) ;
#15563=CARTESIAN_POINT ( 'NONE',  ( 39.44739150791469484, 169.7656965055118974, -43.01277025598062664 ) ) ;
#15565=ORIENTED_EDGE ( 'NONE', *, *, #21009, .T. ) ;
#15572=ORIENTED_EDGE ( 'NONE', *, *, #13061, .T. ) ;
#15577=VERTEX_POINT ( 'NONE', #2099 ) ;
#15585=CARTESIAN_POINT ( 'NONE',  ( 48.54188012090998683, 169.3797848675314128, -113.1351015711598933 ) ) ;
#15586=DIRECTION ( 'NONE',  ( -0.01292394549866739996, -0.005513023399721131770, -0.9999012842304692006 ) ) ;
#15589=EDGE_LOOP ( 'NONE', ( #10239, #6964, #13760, #19185 ) ) ;
#15592=ADVANCED_FACE ( 'NONE', ( #6808 ), #11401, .F. ) ;
#15595=ORIENTED_EDGE ( 'NONE', *, *, #8715, .F. ) ;
#15618=ORIENTED_EDGE ( 'NONE', *, *, #5826, .T. ) ;
#15621=DIRECTION ( 'NONE',  ( -7.125109674161246868E-05, 0.9999848031710253382, -0.005512562950850155054 ) ) ;
#15624=LINE ( 'NONE', #8356, #6220 ) ;
#15627=DIRECTION ( 'NONE',  ( 0.9999164797902015955, 6.965998958219364448E-18, -0.01292414190464157182 ) ) ;
#15630=CARTESIAN_POINT ( 'NONE',  ( -48.58779557229291157, 108.9763022502714591, -43.53992698188888255 ) ) ;
#15631=DIRECTION ( 'NONE',  ( -0.9999164797902015955, -6.965998958219364448E-18, 0.01292414190464157182 ) ) ;
#15633=CARTESIAN_POINT ( 'NONE',  ( 44.31759907479521132, 171.6105373975396162, -53.08687767741515984 ) ) ;
#15636=VERTEX_POINT ( 'NONE', #12562 ) ;
#15648=DIRECTION ( 'NONE',  ( -0.01292394549866736179, -0.005513023399721110954, -0.9999012842304692006 ) ) ;
#15658=ORIENTED_EDGE ( 'NONE', *, *, #6553, .F. ) ;
#15670=SPHERICAL_SURFACE ( 'NONE', #7855, 2.000000000000000000 ) ;
#15678=EDGE_CURVE ( 'NONE', #7828, #9625, #9984, .T. ) ;
#15690=CARTESIAN_POINT ( 'NONE',  ( -40.94813932551374336, 95.97017003981163441, 82.42564028881615457 ) ) ;
#15696=CARTESIAN_POINT ( 'NONE',  ( -51.70139581094897352, 189.5987791479411442, -72.16877407953693080 ) ) ;
#15700=EDGE_CURVE ( 'NONE', #10176, #21136, #6043, .T. ) ;
#15715=VECTOR ( 'NONE', #20549, 1000.000000000000114 ) ;
#15722=DIRECTION ( 'NONE',  ( -7.125109674243555432E-05, 0.9999848031710253382, -0.005512562950850175003 ) ) ;
#15737=DIRECTION ( 'NONE',  ( 0.009371490965938892789, 0.6886276452575282869, 0.7250545781830131098 ) ) ;
#15742=CARTESIAN_POINT ( 'NONE',  ( 14.19652144490156687, 105.7231500355213853, 131.1758847094702389 ) ) ;
#15743=EDGE_CURVE ( 'NONE', #10523, #9499, #2463, .T. ) ;
#15745=DIRECTION ( 'NONE',  ( -7.125109674158749138E-05, 0.9999848031710253382, -0.005512562950850162860 ) ) ;
#15752=CARTESIAN_POINT ( 'NONE',  ( 49.73769616939263472, 110.3486766201082503, -47.52380993751345528 ) ) ;
#15754=DIRECTION ( 'NONE',  ( 7.125109674161259066E-05, -0.9999848031710252272, 0.005512562950850163727 ) ) ;
#15755=DIRECTION ( 'NONE',  ( 0.006595249899610063603, 0.8599936914359664897, 0.5102620438256224578 ) ) ;
#15765=ADVANCED_FACE ( 'NONE', ( #17209 ), #5125, .F. ) ;
#15783=VECTOR ( 'NONE', #20868, 1000.000000000000114 ) ;
#15787=PLANE ( 'NONE',  #18734 ) ;
#15792=ORIENTED_EDGE ( 'NONE', *, *, #12866, .F. ) ;
#15797=CIRCLE ( 'NONE', #10999, 2.000000000000001332 ) ;
#15801=EDGE_LOOP ( 'NONE', ( #21143, #4372, #21892, #15188, #16713, #17249, #1750, #9010, #7570, #4226 ) ) ;
#15802=ORIENTED_EDGE ( 'NONE', *, *, #16282, .F. ) ;
#15820=CARTESIAN_POINT ( 'NONE',  ( -35.42010074854528767, 108.0982075334647163, 199.8475074598744072 ) ) ;
#15821=ORIENTED_EDGE ( 'NONE', *, *, #2370, .F. ) ;
#15823=EDGE_CURVE ( 'NONE', #17283, #7401, #3533, .T. ) ;
#15825=ADVANCED_FACE ( 'NONE', ( #8260 ), #18818, .T. ) ;
#15838=LINE ( 'NONE', #22661, #18314 ) ;
#15839=ORIENTED_EDGE ( 'NONE', *, *, #2852, .T. ) ;
#15841=EDGE_CURVE ( 'NONE', #2746, #21650, #22564, .T. ) ;
#15843=ORIENTED_EDGE ( 'NONE', *, *, #8503, .T. ) ;
#15850=ORIENTED_EDGE ( 'NONE', *, *, #7665, .T. ) ;
#15852=CARTESIAN_POINT ( 'NONE',  ( -10.95317072096182187, 113.6585260871128611, 119.7560427279830009 ) ) ;
#15855=EDGE_CURVE ( 'NONE', #22544, #11891, #13546, .T. ) ;
#15864=DIRECTION ( 'NONE',  ( -0.9999164797902015955, -6.965998958219364448E-18, 0.01292414190464157182 ) ) ;
#15866=DIRECTION ( 'NONE',  ( -0.9999164797902017066, 0.000000000000000000, 0.01292414190463832269 ) ) ;
#15869=PLANE ( 'NONE',  #1337 ) ;
#15873=CARTESIAN_POINT ( 'NONE',  ( 49.97797887564394870, 113.1447607658756880, -44.83689451937377868 ) ) ;
#15891=EDGE_LOOP ( 'NONE', ( #19959, #19281, #245, #11800 ) ) ;
#15904=CARTESIAN_POINT ( 'NONE',  ( 47.42524840967396216, 108.3817487785542824, -44.77763872393808953 ) ) ;
#15910=FACE_OUTER_BOUND ( 'NONE', #21657, .T. ) ;
#15915=EDGE_LOOP ( 'NONE', ( #21597, #6729, #12334, #12501 ) ) ;
#15917=ORIENTED_EDGE ( 'NONE', *, *, #21170, .F. ) ;
#15918=AXIS2_PLACEMENT_3D ( 'NONE', #3253, #17175, #17416 ) ;
#15926=CYLINDRICAL_SURFACE ( 'NONE', #18793, 75.00000000000002842 ) ;
#15930=CARTESIAN_POINT ( 'NONE',  ( -38.77389020828243815, 95.32323862687174199, 83.05169643453594119 ) ) ;
#15941=DIRECTION ( 'NONE',  ( -0.9999164797902017066, 0.000000000000000000, 0.01292414190464157529 ) ) ;
#15958=ORIENTED_EDGE ( 'NONE', *, *, #8572, .F. ) ;
#15980=ORIENTED_EDGE ( 'NONE', *, *, #21684, .F. ) ;
#15984=EDGE_CURVE ( 'NONE', #11891, #16331, #20737, .T. ) ;
#15990=CARTESIAN_POINT ( 'NONE',  ( -48.70980520421279181, 94.99786382055523859, -43.46127891409652477 ) ) ;
#15991=ORIENTED_EDGE ( 'NONE', *, *, #18787, .F. ) ;
#16007=EDGE_CURVE ( 'NONE', #19370, #8189, #16215, .T. ) ;
#16017=ORIENTED_EDGE ( 'NONE', *, *, #4753, .T. ) ;
#16022=CARTESIAN_POINT ( 'NONE',  ( -48.91844876508264406, 94.45452722259994971, 84.00069590936301722 ) ) ;
#16027=DIRECTION ( 'NONE',  ( 0.9999164797902017066, 6.965998958219365988E-18, -0.01292414190464157356 ) ) ;
#16036=DIRECTION ( 'NONE',  ( -7.125109674161259066E-05, 0.9999848031710252272, -0.005512562950850163727 ) ) ;
#16044=CARTESIAN_POINT ( 'NONE',  ( -40.39453254641149726, 94.54797109823962842, 83.85657225284745664 ) ) ;
#16054=ORIENTED_EDGE ( 'NONE', *, *, #9184, .F. ) ;
#16067=ORIENTED_EDGE ( 'NONE', *, *, #4620, .F. ) ;
#16069=CARTESIAN_POINT ( 'NONE',  ( 26.56914632585049674, 169.3906321239456361, -110.8833952302934023 ) ) ;
#16075=LINE ( 'NONE', #5586, #5600 ) ;
#16088=VERTEX_POINT ( 'NONE', #12595 ) ;
#16100=DIRECTION ( 'NONE',  ( 0.9999164797902017066, 6.965998958219365988E-18, -0.01292414190464157356 ) ) ;
#16107=CARTESIAN_POINT ( 'NONE',  ( -51.99565694909051672, 170.0000000000000284, 0.6720553790413400508 ) ) ;
#16110=ADVANCED_FACE ( 'NONE', ( #12251 ), #8896, .T. ) ;
#16121=DIRECTION ( 'NONE',  ( -0.9999164797902015955, -6.965998958219364448E-18, 0.01292414190464157182 ) ) ;
#16137=DIRECTION ( 'NONE',  ( 7.125109674161246868E-05, -0.9999848031710252272, 0.005512562950850154186 ) ) ;
#16146=ADVANCED_FACE ( 'NONE', ( #10750 ), #14736, .T. ) ;
#16150=EDGE_LOOP ( 'NONE', ( #4687, #3562, #3228, #17605 ) ) ;
#16151=CARTESIAN_POINT ( 'NONE',  ( -36.90283430563165723, 95.89798883583559075, 85.13120909300619132 ) ) ;
#16156=CARTESIAN_POINT ( 'NONE',  ( -38.81110560441968715, 96.91202807169366906, 84.24656211158296060 ) ) ;
#16158=CARTESIAN_POINT ( 'NONE',  ( -64.99457118636313169, 170.0000000000000284, 0.8400692238016805868 ) ) ;
#16175=CARTESIAN_POINT ( 'NONE',  ( 14.14224087380716455, 105.6999953372425409, 126.9762993157022777 ) ) ;
#16178=TOROIDAL_SURFACE ( 'NONE', #11765, 85.00000000000000000, 2.000000000000000000 ) ;
#16179=DIRECTION ( 'NONE',  ( -0.01292394549866736873, -0.005513023399721228915, -0.9999012842304690896 ) ) ;
#16180=DIRECTION ( 'NONE',  ( -0.9999164797902015955, -6.965998958219364448E-18, 0.01292414190464157182 ) ) ;
#16188=DIRECTION ( 'NONE',  ( -0.01292394549866738261, -0.005513023399719314648, -0.9999012842304692006 ) ) ;
#16192=AXIS2_PLACEMENT_3D ( 'NONE', #21408, #8765, #7180 ) ;
#16202=VECTOR ( 'NONE', #3824, 999.9999999999998863 ) ;
#16204=DIRECTION ( 'NONE',  ( -7.125109674161242803E-05, 0.9999848031710252272, -0.005512562950850150717 ) ) ;
#16215=CIRCLE ( 'NONE', #16923, 1.999999999999999778 ) ;
#16217=CARTESIAN_POINT ( 'NONE',  ( -50.54267232652800601, 95.91485852618909291, -44.96266421069820041 ) ) ;
#16218=ORIENTED_EDGE ( 'NONE', *, *, #10520, .F. ) ;
#16221=CARTESIAN_POINT ( 'NONE',  ( 51.99565694909048830, 170.0000000000000284, -0.6720553790413839046 ) ) ;
#16223=CARTESIAN_POINT ( 'NONE',  ( -42.42378443038275293, 94.99786382055523859, -43.54252712446056961 ) ) ;
#16251=VECTOR ( 'NONE', #1130, 1000.000000000000000 ) ;
#16268=EDGE_CURVE ( 'NONE', #17449, #22622, #1161, .T. ) ;
#16273=CARTESIAN_POINT ( 'NONE',  ( -39.54589198439538933, 93.83276874622022490, 84.56879583056640115 ) ) ;
#16276=CARTESIAN_POINT ( 'NONE',  ( 45.19575868936945540, 125.3640259171584290, 246.9784031832207631 ) ) ;
#16282=EDGE_CURVE ( 'NONE', #10034, #16304, #9354, .T. ) ;
#16286=EDGE_CURVE ( 'NONE', #719, #22322, #5906, .T. ) ;
#16287=AXIS2_PLACEMENT_3D ( 'NONE', #5341, #302, #9014 ) ;
#16298=DIRECTION ( 'NONE',  ( -0.01292394549866737914, -0.005513023399721009472, -0.9999012842304692006 ) ) ;
#16304=VERTEX_POINT ( 'NONE', #11208 ) ;
#16306=CARTESIAN_POINT ( 'NONE',  ( 14.13996083871143306, 137.6995090387153482, 126.7998973012750810 ) ) ;
#16310=CARTESIAN_POINT ( 'NONE',  ( 41.18784844526823719, 107.5071733437152375, 91.64309988731913847 ) ) ;
#16318=ORIENTED_EDGE ( 'NONE', *, *, #6323, .F. ) ;
#16322=ORIENTED_EDGE ( 'NONE', *, *, #11932, .T. ) ;
#16331=VERTEX_POINT ( 'NONE', #1435 ) ;
#16336=ORIENTED_EDGE ( 'NONE', *, *, #15162, .F. ) ;
#16337=EDGE_LOOP ( 'NONE', ( #9539, #14371, #257, #18042 ) ) ;
#16339=DIRECTION ( 'NONE',  ( -0.01292394549866736179, -0.005513023399721110954, -0.9999012842304692006 ) ) ;
#16340=CARTESIAN_POINT ( 'NONE',  ( -40.78795384167224825, 95.60340320854591312, -42.51611673894687016 ) ) ;
#16343=DIRECTION ( 'NONE',  ( -0.9999164797902015955, -6.965998958219364448E-18, 0.01292414190464157182 ) ) ;
#16345=CARTESIAN_POINT ( 'NONE',  ( 45.22132157597982882, 129.3749911766419700, 248.9561554998783208 ) ) ;
#16348=CARTESIAN_POINT ( 'NONE',  ( 42.78098668172552976, 106.8060942374655156, 70.38625157530108822 ) ) ;
#16349=FACE_OUTER_BOUND ( 'NONE', #18478, .T. ) ;
#16356=ORIENTED_EDGE ( 'NONE', *, *, #10021, .F. ) ;
#16366=CARTESIAN_POINT ( 'NONE',  ( 50.04172213657920310, 189.5996388551388918, -73.32787460386838063 ) ) ;
#16371=CARTESIAN_POINT ( 'NONE',  ( 53.22133760583491124, 119.7725967263615985, 248.9056969729654440 ) ) ;
#16372=CARTESIAN_POINT ( 'NONE',  ( 39.89762790624313737, 105.6320600527179607, 91.75806838212221805 ) ) ;
#16375=AXIS2_PLACEMENT_3D ( 'NONE', #9523, #17007, #6311 ) ;
#16380=ORIENTED_EDGE ( 'NONE', *, *, #14566, .F. ) ;
#16389=EDGE_CURVE ( 'NONE', #2091, #19509, #5549, .T. ) ;
#16393=DIRECTION ( 'NONE',  ( -0.9999164797902015955, -6.965998958219364448E-18, 0.01292414190464157182 ) ) ;
#16396=CARTESIAN_POINT ( 'NONE',  ( 49.22751544813647939, 112.6450176187863832, -44.82443924574226202 ) ) ;
#16397=FACE_OUTER_BOUND ( 'NONE', #5669, .T. ) ;
#16402=CYLINDRICAL_SURFACE ( 'NONE', #8876, 112.5000000000000142 ) ;
#16404=DIRECTION ( 'NONE',  ( 0.9999164797902015955, 6.965998958219364448E-18, -0.01292414190464157182 ) ) ;
#16417=B_SPLINE_CURVE_WITH_KNOTS ( 'NONE', 3,
 ( #21983, #21867, #7775, #4309, #1121, #18463, #4543, #5932, #21760, #18239, #11570, #20051, #1004, #16650, #18570, #19936 ),
 .UNSPECIFIED., .F., .F.,
 ( 4, 2, 2, 2, 2, 2, 2, 4 ),
 ( 0.000000000000000000, 0.0003951513861477968419, 0.0007903027722955936838, 0.001185454158443390634, 0.001580605544591187368, 0.001975756930738984101, 0.002370908316886781268, 0.003161211089182393817 ),
 .UNSPECIFIED. ) ;
#16420=DIRECTION ( 'NONE',  ( -0.9999164797902017066, 0.000000000000000000, 0.01292414190463832269 ) ) ;
#16422=CIRCLE ( 'NONE', #4277, 112.5000000000007105 ) ;
#16435=VERTEX_POINT ( 'NONE', #1328 ) ;
#16454=CYLINDRICAL_SURFACE ( 'NONE', #10605, 102.6746853779045381 ) ;
#16464=ORIENTED_EDGE ( 'NONE', *, *, #62, .F. ) ;
#16474=EDGE_CURVE ( 'NONE', #5966, #7339, #19487, .T. ) ;
#16475=CARTESIAN_POINT ( 'NONE',  ( 39.48249285872903158, 105.5238643664723668, 91.68783210470924416 ) ) ;
#16478=DIRECTION ( 'NONE',  ( -0.9999164797902015955, -6.965998958219364448E-18, 0.01292414190464157182 ) ) ;
#16482=ORIENTED_EDGE ( 'NONE', *, *, #7665, .F. ) ;
#16501=TOROIDAL_SURFACE ( 'NONE', #13548, 93.00000000000000000, 2.000000000000000000 ) ;
#16502=ORIENTED_EDGE ( 'NONE', *, *, #19417, .T. ) ;
#16510=DIRECTION ( 'NONE',  ( 0.01292394549866739996, 0.005513023399721131770, 0.9999012842304692006 ) ) ;
#16528=ORIENTED_EDGE ( 'NONE', *, *, #5826, .F. ) ;
#16531=VERTEX_POINT ( 'NONE', #21054 ) ;
#16542=AXIS2_PLACEMENT_3D ( 'NONE', #19374, #11121, #3969 ) ;
#16545=CARTESIAN_POINT ( 'NONE',  ( 40.93042701181084908, 108.3156947416822362, 71.72688916598494302 ) ) ;
#16560=AXIS2_PLACEMENT_3D ( 'NONE', #2158, #15745, #15866 ) ;
#16569=LINE ( 'NONE', #13112, #3245 ) ;
#16571=CARTESIAN_POINT ( 'NONE',  ( -51.19659413568783890, 110.8744609730857178, -46.41152423219341472 ) ) ;
#16576=DIRECTION ( 'NONE',  ( 0.9999164797902015955, 6.965998958219364448E-18, -0.01292414190464157182 ) ) ;
#16579=FACE_OUTER_BOUND ( 'NONE', #2100, .T. ) ;
#16585=CARTESIAN_POINT ( 'NONE',  ( -45.96195738621045024, 164.6879759653328961, -74.13402305205957532 ) ) ;
#16589=EDGE_CURVE ( 'NONE', #10697, #12374, #20934, .T. ) ;
#16593=CARTESIAN_POINT ( 'NONE',  ( -50.86956732378053658, 110.1619587132339717, -46.15522227794017596 ) ) ;
#16594=ORIENTED_EDGE ( 'NONE', *, *, #5452, .F. ) ;
#16603=CARTESIAN_POINT ( 'NONE',  ( -50.56692998826083851, 113.4816418249608034, -43.53918672598639716 ) ) ;
#16614=ORIENTED_EDGE ( 'NONE', *, *, #16474, .F. ) ;
#16615=DIRECTION ( 'NONE',  ( 0.9999164797902015955, 6.965998958219364448E-18, -0.01292414190464157182 ) ) ;
#16617=VECTOR ( 'NONE', #17949, 1000.000000000000114 ) ;
#16619=DIRECTION ( 'NONE',  ( 0.01292394549866740169, 0.005513023399720822990, 0.9999012842304693116 ) ) ;
#16624=DIRECTION ( 'NONE',  ( -0.01292394549866741904, -0.005513023399721091004, -0.9999012842304693116 ) ) ;
#16628=CIRCLE ( 'NONE', #3014, 93.00000000000001421 ) ;
#16629=CARTESIAN_POINT ( 'NONE',  ( 41.17443399381281921, 107.5575245709146941, 71.06985290734100147 ) ) ;
#16631=EDGE_CURVE ( 'NONE', #13286, #848, #18408, .T. ) ;
#16636=CARTESIAN_POINT ( 'NONE',  ( 40.57355171551004247, 108.0982075334647163, 198.8652726751216733 ) ) ;
#16638=CARTESIAN_POINT ( 'NONE',  ( -64.22027802397437313, 106.9149828242082947, 60.74567061489647557 ) ) ;
#16649=ORIENTED_EDGE ( 'NONE', *, *, #8921, .F. ) ;
#16650=CARTESIAN_POINT ( 'NONE',  ( 50.26215390436148311, 189.4880035784398160, -93.58148208147835589 ) ) ;
#16651=CARTESIAN_POINT ( 'NONE',  ( 64.31784532510161512, 144.7109461922390778, -53.19707257213011076 ) ) ;
#16656=VECTOR ( 'NONE', #13511, 1000.000000000000000 ) ;
#16681=CARTESIAN_POINT ( 'NONE',  ( -39.24016587203285411, 108.3652131041115467, 59.04542680541619859 ) ) ;
#16690=EDGE_CURVE ( 'NONE', #22542, #17948, #7035, .T. ) ;
#16691=CARTESIAN_POINT ( 'NONE',  ( -50.82071652507229231, 109.9724431479075832, -46.08693180671795631 ) ) ;
#16712=VERTEX_POINT ( 'NONE', #17139 ) ;
#16713=ORIENTED_EDGE ( 'NONE', *, *, #14129, .T. ) ;
#16717=ADVANCED_FACE ( 'NONE', ( #13806 ), #15430, .F. ) ;
#16722=CARTESIAN_POINT ( 'NONE',  ( -38.19275834114522894, 94.78920923681313582, 83.58418063251983199 ) ) ;
#16723=ORIENTED_EDGE ( 'NONE', *, *, #9480, .T. ) ;
#16724=DIRECTION ( 'NONE',  ( 0.9999164797902015955, 6.965998958219364448E-18, -0.01292414190464157182 ) ) ;
#16730=ADVANCED_FACE ( 'NONE', ( #11971 ), #22268, .T. ) ;
#16733=ORIENTED_EDGE ( 'NONE', *, *, #3358, .T. ) ;
#16737=CARTESIAN_POINT ( 'NONE',  ( -41.15169610061244754, 101.1708071963161615, 65.90309081746964637 ) ) ;
#16738=VERTEX_POINT ( 'NONE', #4701 ) ;
#16740=EDGE_CURVE ( 'NONE', #2396, #17033, #4796, .T. ) ;
#16744=CARTESIAN_POINT ( 'NONE',  ( -39.99665919160808869, 170.0000000000000284, 0.5169656761856410432 ) ) ;
#16767=ORIENTED_EDGE ( 'NONE', *, *, #11932, .F. ) ;
#16769=DIRECTION ( 'NONE',  ( -0.01292394549866695240, -0.005513023399725255208, -0.9999012842304693116 ) ) ;
#16771=ORIENTED_EDGE ( 'NONE', *, *, #19305, .T. ) ;
#16782=CARTESIAN_POINT ( 'NONE',  ( -35.42010074854528767, 108.0982075334647163, 199.8475074598744357 ) ) ;
#16786=ADVANCED_FACE ( 'NONE', ( #8287 ), #15320, .F. ) ;
#16808=DIRECTION ( 'NONE',  ( 0.01292394549866705648, 0.005513023399720703294, 0.9999012842304692006 ) ) ;
#16821=DIRECTION ( 'NONE',  ( -0.01292394549866740343, -0.005513023399721215904, -0.9999012842304693116 ) ) ;
#16825=LINE ( 'NONE', #1207, #4166 ) ;
#16847=EDGE_CURVE ( 'NONE', #17590, #1849, #9291, .T. ) ;
#16850=CARTESIAN_POINT ( 'NONE',  ( 42.43719399169239637, 94.56237283683982753, 82.91753452609758313 ) ) ;
#16859=ORIENTED_EDGE ( 'NONE', *, *, #14984, .F. ) ;
#16864=ORIENTED_EDGE ( 'NONE', *, *, #18428, .T. ) ;
#16874=DIRECTION ( 'NONE',  ( -7.125109674243555432E-05, 0.9999848031710253382, -0.005512562950850175003 ) ) ;
#16887=CIRCLE ( 'NONE', #3295, 110.5324305509042233 ) ;
#16891=CARTESIAN_POINT ( 'NONE',  ( 42.92324425022518852, 106.8061942917681790, 70.38450200964520320 ) ) ;
#16892=FACE_OUTER_BOUND ( 'NONE', #17089, .T. ) ;
#16893=ORIENTED_EDGE ( 'NONE', *, *, #511, .F. ) ;
#16902=AXIS2_PLACEMENT_3D ( 'NONE', #7260, #12449, #13832 ) ;
#16909=( BOUNDED_CURVE ( )  B_SPLINE_CURVE ( 3, ( #7802, #9646, #4333, #21461 ),
 .UNSPECIFIED., .F., .T. ) 
 B_SPLINE_CURVE_WITH_KNOTS ( ( 4, 4 ),
 ( 3.141592653589793560, 4.712388980384689674 ),
 .UNSPECIFIED. ) 
 CURVE ( )  GEOMETRIC_REPRESENTATION_ITEM ( )  RATIONAL_B_SPLINE_CURVE ( ( 1.000000000000000000, 0.8047378541243650485, 0.8047378541243650485, 1.000000000000000000 ) ) 
 REPRESENTATION_ITEM ( '' )  );
#16911=ORIENTED_EDGE ( 'NONE', *, *, #169, .F. ) ;
#16923=AXIS2_PLACEMENT_3D ( 'NONE', #15820, #10967, #12371 ) ;
#16934=DIRECTION ( 'NONE',  ( -0.01292394549866743465, -0.005513023399721021615, -0.9999012842304692006 ) ) ;
#16936=B_SPLINE_CURVE_WITH_KNOTS ( 'NONE', 3,
 ( #2342, #21499, #14309, #18204, #7613, #12798, #19772, #4047, #2452, #11072, #9447, #14651, #19447, #10733, #17762, #2006 ),
 .UNSPECIFIED., .F., .F.,
 ( 4, 2, 2, 2, 2, 2, 2, 4 ),
 ( -9.611261265246428336E-06, 0.0004115787608243976327, 0.0008327687829140417632, 0.001253958805003685568, 0.001675148827093329807, 0.002517528871272620237, 0.002938718893362260356, 0.003359908915451900908 ),
 .UNSPECIFIED. ) ;
#16943=DIRECTION ( 'NONE',  ( 0.003413786507422414233, -0.9644842718275420390, 0.2641182225045781706 ) ) ;
#16944=CARTESIAN_POINT ( 'NONE',  ( -40.94813932551373625, 95.97017003981163441, 82.42564028881616878 ) ) ;
#16947=DIRECTION ( 'NONE',  ( -0.9999164797902015955, -6.965998958219364448E-18, 0.01292414190464157182 ) ) ;
#16957=ORIENTED_EDGE ( 'NONE', *, *, #8252, .T. ) ;
#16958=CARTESIAN_POINT ( 'NONE',  ( -21.67182210555940358, 59.11803865240464262, -129.2164758598523235 ) ) ;
#16961=EDGE_LOOP ( 'NONE', ( #12402, #20497, #6304, #7453 ) ) ;
#16963=DIRECTION ( 'NONE',  ( -0.9999164797902015955, -6.965998958219364448E-18, 0.01292414190464157182 ) ) ;
#16964=CARTESIAN_POINT ( 'NONE',  ( -50.43108932508832964, 106.8786590446587184, 71.51684434343255248 ) ) ;
#16970=LINE ( 'NONE', #1231, #16656 ) ;
#16973=DIRECTION ( 'NONE',  ( 0.01292394549866740169, 0.005513023399720822990, 0.9999012842304693116 ) ) ;
#16974=CARTESIAN_POINT ( 'NONE',  ( 43.08423624159371457, 94.48610424851698042, 82.84014869562157912 ) ) ;
#16975=CARTESIAN_POINT ( 'NONE',  ( -64.99457118636313169, 170.0000000000000284, 0.8400692238016805868 ) ) ;
#16977=EDGE_CURVE ( 'NONE', #21004, #17590, #8138, .T. ) ;
#16981=AXIS2_PLACEMENT_3D ( 'NONE', #21994, #8334, #22326 ) ;
#16998=ADVANCED_FACE ( 'NONE', ( #22452 ), #17202, .T. ) ;
#17003=CARTESIAN_POINT ( 'NONE',  ( -36.90283430563165723, 95.89798883583559075, 85.13120909300619132 ) ) ;
#17007=DIRECTION ( 'NONE',  ( 0.9999164797902017066, 6.965998958219365988E-18, -0.01292414190464157356 ) ) ;
#17008=CARTESIAN_POINT ( 'NONE',  ( 64.42123688909094881, 144.7550503794368524, -45.19786229828635271 ) ) ;
#17018=TOROIDAL_SURFACE ( 'NONE', #12619, 4.000000000000000000, 2.000000000000000000 ) ;
#17020=CARTESIAN_POINT ( 'NONE',  ( -51.88617280806869303, 111.6760431855662716, -46.69719173690569392 ) ) ;
#17025=DIRECTION ( 'NONE',  ( -0.01292394549866739996, -0.005513023399721131770, -0.9999012842304692006 ) ) ;
#17028=ORIENTED_EDGE ( 'NONE', *, *, #12573, .T. ) ;
#17033=VERTEX_POINT ( 'NONE', #22231 ) ;
#17037=ORIENTED_EDGE ( 'NONE', *, *, #3449, .F. ) ;
#17038=CARTESIAN_POINT ( 'NONE',  ( 48.49194500006319686, 95.17841068403271265, -45.02347578433171549 ) ) ;
#17049=DIRECTION ( 'NONE',  ( 0.01292394549866739822, 0.005513023399721908059, 0.9999012842304692006 ) ) ;
#17054=CARTESIAN_POINT ( 'NONE',  ( -51.96399215116387182, 189.4900423377766003, -91.89035338882484893 ) ) ;
#17074=AXIS2_PLACEMENT_3D ( 'NONE', #16782, #20318, #20529 ) ;
#17076=CARTESIAN_POINT ( 'NONE',  ( -51.07890516687701421, 106.8060942374655156, 71.59941146007480484 ) ) ;
#17080=DIRECTION ( 'NONE',  ( -0.9999164797902017066, -6.965998958219365988E-18, 0.01292414190464157356 ) ) ;
#17089=EDGE_LOOP ( 'NONE', ( #21926, #23, #4703, #22178 ) ) ;
#17093=DIRECTION ( 'NONE',  ( -0.01292394549866740690, -0.005513023399721241925, -0.9999012842304693116 ) ) ;
#17103=EDGE_CURVE ( 'NONE', #2719, #10523, #9261, .T. ) ;
#17113=LINE ( 'NONE', #4910, #15783 ) ;
#17119=DIRECTION ( 'NONE',  ( 7.125109674161246868E-05, -0.9999848031710253382, 0.005512562950850155054 ) ) ;
#17125=VERTEX_POINT ( 'NONE', #21530 ) ;
#17127=CARTESIAN_POINT ( 'NONE',  ( 49.43718378874159214, 109.1839087875310810, -47.09652170433833618 ) ) ;
#17130=DIRECTION ( 'NONE',  ( 7.125109674161246868E-05, -0.9999848031710253382, 0.005512562950850155054 ) ) ;
#17132=DIRECTION ( 'NONE',  ( -0.01096700916508639573, 0.5290868411612598132, -0.8484968115555726609 ) ) ;
#17137=CARTESIAN_POINT ( 'NONE',  ( 47.98905872121961380, 95.04270968059627478, -44.78735749829896662 ) ) ;
#17139=CARTESIAN_POINT ( 'NONE',  ( 41.42670316190684332, 94.99786382055523859, -44.62631324292065926 ) ) ;
#17140=ORIENTED_EDGE ( 'NONE', *, *, #9222, .F. ) ;
#17147=CARTESIAN_POINT ( 'NONE',  ( 49.46148465141350670, 112.8301064087732897, -44.82848384907012473 ) ) ;
#17148=CIRCLE ( 'NONE', #19335, 7.921742784567035400 ) ;
#17149=CARTESIAN_POINT ( 'NONE',  ( -53.19734013806819206, 189.4876967392748384, -92.29990616481009624 ) ) ;
#17155=CARTESIAN_POINT ( 'NONE',  ( -42.56982644846065966, 144.7550503794368524, -43.81497911448970228 ) ) ;
#17166=CARTESIAN_POINT ( 'NONE',  ( 50.84062004008612234, 101.1708071963161615, 64.71406976224261598 ) ) ;
#17169=EDGE_LOOP ( 'NONE', ( #22585, #16733, #21899, #7847 ) ) ;
#17170=CARTESIAN_POINT ( 'NONE',  ( -65.56567718511387000, 113.4816418249608034, -43.34532459741677002 ) ) ;
#17171=DIRECTION ( 'NONE',  ( 0.01292394549866738782, 0.005513023399721118760, 0.9999012842304692006 ) ) ;
#17175=DIRECTION ( 'NONE',  ( 0.9999164797902017066, 6.965998958219367529E-18, -0.01292414190464157182 ) ) ;
#17178=CARTESIAN_POINT ( 'NONE',  ( 41.09169241204631362, 95.99012513974443550, 84.20368898025243709 ) ) ;
#17180=CARTESIAN_POINT ( 'NONE',  ( -51.04847592823571034, 189.5933835232740989, -73.15598528727107919 ) ) ;
#17195=ORIENTED_EDGE ( 'NONE', *, *, #18352, .F. ) ;
#17202=CYLINDRICAL_SURFACE ( 'NONE', #2281, 110.5324305509042233 ) ;
#17203=EDGE_CURVE ( 'NONE', #2844, #22542, #16628, .T. ) ;
#17208=CARTESIAN_POINT ( 'NONE',  ( 64.99770623461974139, 126.0006686604749291, -0.5975164539643176287 ) ) ;
#17209=FACE_OUTER_BOUND ( 'NONE', #18219, .T. ) ;
#17221=DIRECTION ( 'NONE',  ( -0.01292394549866772609, -0.005513023399720218438, -0.9999012842304693116 ) ) ;
#17222=FACE_OUTER_BOUND ( 'NONE', #16961, .T. ) ;
#17229=DIRECTION ( 'NONE',  ( 0.01292394549866740169, 0.005513023399721131770, 0.9999012842304693116 ) ) ;
#17232=CARTESIAN_POINT ( 'NONE',  ( 49.61333693951482360, 109.9750644004051594, -47.38601841831088990 ) ) ;
#17235=EDGE_CURVE ( 'NONE', #19636, #956, #20622, .T. ) ;
#17236=DIRECTION ( 'NONE',  ( -0.9999164797902015955, -6.965998958219364448E-18, 0.01292414190464157182 ) ) ;
#17237=DIRECTION ( 'NONE',  ( -0.9999164797902015955, -6.965998958219364448E-18, 0.01292414190464157182 ) ) ;
#17245=ORIENTED_EDGE ( 'NONE', *, *, #9701, .T. ) ;
#17248=DIRECTION ( 'NONE',  ( 7.125109674161246868E-05, -0.9999848031710252272, 0.005512562950850154186 ) ) ;
#17249=ORIENTED_EDGE ( 'NONE', *, *, #20579, .T. ) ;
#17258=DIRECTION ( 'NONE',  ( 0.01292394549866695240, 0.005513023399725255208, 0.9999012842304693116 ) ) ;
#17272=CARTESIAN_POINT ( 'NONE',  ( -40.94471193931616426, 95.70788552361970858, 82.69081069369302384 ) ) ;
#17279=VECTOR ( 'NONE', #16963, 1000.000000000000000 ) ;
#17282=ORIENTED_EDGE ( 'NONE', *, *, #532, .T. ) ;
#17283=VERTEX_POINT ( 'NONE', #15226 ) ;
#17284=DIRECTION ( 'NONE',  ( -0.01292394549866740343, -0.005513023399721215904, -0.9999012842304693116 ) ) ;
#17285=EDGE_CURVE ( 'NONE', #552, #6085, #6236, .T. ) ;
#17287=EDGE_CURVE ( 'NONE', #9119, #9213, #12576, .T. ) ;
#17293=CARTESIAN_POINT ( 'NONE',  ( -64.99457118636311748, 170.0000000000008242, 0.8400692238025471159 ) ) ;
#17295=FACE_OUTER_BOUND ( 'NONE', #5994, .T. ) ;
#17297=CARTESIAN_POINT ( 'NONE',  ( 42.19468217728159942, 94.63733313072589226, 82.98836926700062122 ) ) ;
#17298=DIRECTION ( 'NONE',  ( -0.9999164797902017066, 0.000000000000000000, 0.01292414190464157529 ) ) ;
#17303=VECTOR ( 'NONE', #2358, 1000.000000000000114 ) ;
#17306=ORIENTED_EDGE ( 'NONE', *, *, #14129, .F. ) ;
#17321=ORIENTED_EDGE ( 'NONE', *, *, #4440, .T. ) ;
#17323=CARTESIAN_POINT ( 'NONE',  ( 64.31884524158141403, 144.7109461922390778, -53.19708549627201677 ) ) ;
#17345=DIRECTION ( 'NONE',  ( 0.9999164797902015955, 6.965998958219364448E-18, -0.01292414190464157182 ) ) ;
#17352=EDGE_LOOP ( 'NONE', ( #20056, #3210, #2444 ) ) ;
#17375=TOROIDAL_SURFACE ( 'NONE', #21030, 9.921742784567035400, 2.000000000000000000 ) ;
#17379=CIRCLE ( 'NONE', #136, 1.999999999999999778 ) ;
#17380=ORIENTED_EDGE ( 'NONE', *, *, #17685, .F. ) ;
#17382=CARTESIAN_POINT ( 'NONE',  ( 43.19621557115664245, 121.2962013336460956, 247.0266759469006672 ) ) ;
#17386=CARTESIAN_POINT ( 'NONE',  ( 19.42556530730579567, 136.7551719540686008, -44.57217540897067920 ) ) ;
#17391=DIRECTION ( 'NONE',  ( -7.125109674161231961E-05, 0.9999848031710252272, -0.005512562950850142043 ) ) ;
#17395=CARTESIAN_POINT ( 'NONE',  ( -65.56655171279719241, 125.7553391191873544, -43.41298515461679131 ) ) ;
#17402=VECTOR ( 'NONE', #17345, 1000.000000000000000 ) ;
#17404=ORIENTED_EDGE ( 'NONE', *, *, #1139, .F. ) ;
#17405=ORIENTED_EDGE ( 'NONE', *, *, #21105, .F. ) ;
#17409=ORIENTED_EDGE ( 'NONE', *, *, #7532, .F. ) ;
#17416=DIRECTION ( 'NONE',  ( -0.01292394549866739996, -0.005513023399721131770, -0.9999012842304692006 ) ) ;
#17422=FACE_OUTER_BOUND ( 'NONE', #6811, .T. ) ;
#17426=CARTESIAN_POINT ( 'NONE',  ( -38.16002667504573509, 95.06337575508095483, 84.40961337517086349 ) ) ;
#17428=ORIENTED_EDGE ( 'NONE', *, *, #20194, .T. ) ;
#17442=PLANE ( 'NONE',  #7496 ) ;
#17447=ADVANCED_FACE ( 'NONE', ( #15361 ), #1557, .F. ) ;
#17449=VERTEX_POINT ( 'NONE', #15585 ) ;
#17471=CARTESIAN_POINT ( 'NONE',  ( -49.41143953161469682, 111.5125656627889015, -43.54326506131044994 ) ) ;
#17478=CARTESIAN_POINT ( 'NONE',  ( 51.38234815825343560, 111.9218655255082382, -48.12259961501337102 ) ) ;
#17485=CARTESIAN_POINT ( 'NONE',  ( 28.96536656690224021, 99.74539563421257071, 74.50764472524521409 ) ) ;
#17492=DIRECTION ( 'NONE',  ( 0.01292394549866737220, 0.005513023399721000799, 0.9999012842304692006 ) ) ;
#17497=CYLINDRICAL_SURFACE ( 'NONE', #6001, 102.6746853779045381 ) ;
#17499=ORIENTED_EDGE ( 'NONE', *, *, #17786, .T. ) ;
#17504=EDGE_CURVE ( 'NONE', #2673, #14965, #14322, .T. ) ;
#17519=AXIS2_PLACEMENT_3D ( 'NONE', #18037, #9286, #21552 ) ;
#17521=FACE_OUTER_BOUND ( 'NONE', #22497, .T. ) ;
#17524=CARTESIAN_POINT ( 'NONE',  ( -40.94568735521033886, 95.78253051705814869, 82.61534438928066493 ) ) ;
#17553=DIRECTION ( 'NONE',  ( -0.9999164797902015955, -6.965998958219364448E-18, 0.01292414190464157182 ) ) ;
#17555=CARTESIAN_POINT ( 'NONE',  ( 50.89493962932122173, 107.8908830597778064, 68.91667391595403558 ) ) ;
#17576=CARTESIAN_POINT ( 'NONE',  ( -50.73053929929668726, 108.7816493830516151, -43.51115831301089543 ) ) ;
#17578=DIRECTION ( 'NONE',  ( -0.01292394549866743465, -0.005513023399721021615, -0.9999012842304692006 ) ) ;
#17582=FACE_OUTER_BOUND ( 'NONE', #10701, .T. ) ;
#17586=VERTEX_POINT ( 'NONE', #3938 ) ;
#17590=VERTEX_POINT ( 'NONE', #6126 ) ;
#17591=LINE ( 'NONE', #3331, #2701 ) ;
#17598=CARTESIAN_POINT ( 'NONE',  ( -65.67129704762463405, 144.7109461922390778, -51.51693412452669918 ) ) ;
#17605=ORIENTED_EDGE ( 'NONE', *, *, #4609, .F. ) ;
#17620=ORIENTED_EDGE ( 'NONE', *, *, #20725, .F. ) ;
#17622=ORIENTED_EDGE ( 'NONE', *, *, #13196, .T. ) ;
#17632=CYLINDRICAL_SURFACE ( 'NONE', #19737, 2.000000000000001332 ) ;
#17633=DIRECTION ( 'NONE',  ( 0.9999164797902017066, 6.965998958219365988E-18, -0.01292414190464157356 ) ) ;
#17637=CARTESIAN_POINT ( 'NONE',  ( -38.94547111459952760, 95.87640844880095869, 82.49456443487720492 ) ) ;
#17641=DIRECTION ( 'NONE',  ( 0.9999164797902015955, 6.965998958219364448E-18, -0.01292414190464157182 ) ) ;
#17644=EDGE_CURVE ( 'NONE', #20719, #19509, #16887, .T. ) ;
#17656=ORIENTED_EDGE ( 'NONE', *, *, #22228, .F. ) ;
#17659=EDGE_CURVE ( 'NONE', #18018, #2060, #9228, .T. ) ;
#17666=ORIENTED_EDGE ( 'NONE', *, *, #11361, .F. ) ;
#17678=ORIENTED_EDGE ( 'NONE', *, *, #451, .T. ) ;
#17681=CARTESIAN_POINT ( 'NONE',  ( 44.03052579490771024, 164.6879759653328961, -75.29719582347730977 ) ) ;
#17685=EDGE_CURVE ( 'NONE', #3794, #6936, #20116, .T. ) ;
#17693=CARTESIAN_POINT ( 'NONE',  ( 49.42384346307601106, 125.7553391191873544, -44.89926147365057574 ) ) ;
#17694=EDGE_CURVE ( 'NONE', #2170, #6548, #18698, .T. ) ;
#17696=VECTOR ( 'NONE', #22123, 1000.000000000000114 ) ;
#17701=VECTOR ( 'NONE', #6653, 1000.000000000000000 ) ;
#17704=CARTESIAN_POINT ( 'NONE',  ( -51.12457683484994675, 113.1366485501290953, -43.53007687325056452 ) ) ;
#17715=DIRECTION ( 'NONE',  ( -0.01292394549866740863, -0.005513023399721009472, -0.9999012842304692006 ) ) ;
#17717=VECTOR ( 'NONE', #20996, 999.9999999999998863 ) ;
#17718=AXIS2_PLACEMENT_3D ( 'NONE', #9367, #19801, #16934 ) ;
#17727=CARTESIAN_POINT ( 'NONE',  ( -36.80549447617401881, 105.5072037373731888, 92.66220808178287882 ) ) ;
#17734=B_SPLINE_CURVE_WITH_KNOTS ( 'NONE', 3,
 ( #10117, #15525, #22478, #4473, #7222, #22584, #5514, #10801, #17471, #6993, #3318, #3441, #14143, #3657, #17704, #5030, #12064, #13897, #14251, #3779 ),
 .UNSPECIFIED., .F., .F.,
 ( 4, 2, 2, 2, 2, 2, 2, 2, 2, 4 ),
 ( 0.000000000000000000, 0.0008942227389302294686, 0.001788445477860458937, 0.002682668216790688731, 0.003576890955720917874, 0.004471113694651147018, 0.005365336433581377462, 0.005812447803046480975, 0.006259559172511584488, 0.007153781911441802789 ),
 .UNSPECIFIED. ) ;
#17741=DIRECTION ( 'NONE',  ( -0.9999164797902015955, -6.965998958219364448E-18, 0.01292414190464157182 ) ) ;
#17756=ORIENTED_EDGE ( 'NONE', *, *, #1984, .T. ) ;
#17762=CARTESIAN_POINT ( 'NONE',  ( 41.28420658616847305, 94.99786382055521017, -44.62447144312741898 ) ) ;
#17767=CARTESIAN_POINT ( 'NONE',  ( -38.64445966580888836, 96.64268400674895076, 84.48542380140278851 ) ) ;
#17777=VERTEX_POINT ( 'NONE', #13387 ) ;
#17778=VECTOR ( 'NONE', #3688, 1000.000000000000000 ) ;
#17786=EDGE_CURVE ( 'NONE', #3794, #15416, #21616, .T. ) ;
#17787=DIRECTION ( 'NONE',  ( 7.125109674161246868E-05, -0.9999848031710252272, 0.005512562950850154186 ) ) ;
#17789=CARTESIAN_POINT ( 'NONE',  ( 44.31759907479521132, 171.6105373975396162, -53.08687767741515984 ) ) ;
#17795=VECTOR ( 'NONE', #13659, 1000.000000000000000 ) ;
#17803=ORIENTED_EDGE ( 'NONE', *, *, #10203, .T. ) ;
#17807=ADVANCED_FACE ( 'NONE', ( #8302 ), #15335, .T. ) ;
#17813=COLOUR_RGB ( '', 0.31764706, 0.68627451, 0.89019608) ;
#17818=EDGE_CURVE ( 'NONE', #7542, #5831, #3130, .T. ) ;
#17820=CARTESIAN_POINT ( 'NONE',  ( 50.14582690138693977, 111.1418060336978186, -47.81946391486589931 ) ) ;
#17825=VERTEX_POINT ( 'NONE', #9916 ) ;
#17839=B_SPLINE_CURVE_WITH_KNOTS ( 'NONE', 3,
 ( #14468, #8788, #21433, #14114, #21529, #10536, #3961, #548, #19366, #14228, #5348, #9138, #17555, #1803 ),
 .UNSPECIFIED., .F., .F.,
 ( 4, 2, 2, 2, 2, 2, 4 ),
 ( 0.000000000000000000, 0.0003918831267809858715, 0.0007837662535619717430, 0.001175649380342957831, 0.001567532507123943486, 0.002351298760685859284, 0.003135065014247775082 ),
 .UNSPECIFIED. ) ;
#17845=ORIENTED_EDGE ( 'NONE', *, *, #1069, .F. ) ;
#17858=DIRECTION ( 'NONE',  ( 0.01292394549866739996, 0.005513023399721131770, 0.9999012842304692006 ) ) ;
#17863=CARTESIAN_POINT ( 'NONE',  ( -39.85606267361366406, 107.1132303434984578, 71.72685069023916071 ) ) ;
#17871=PLANE ( 'NONE',  #2368 ) ;
#17873=EDGE_CURVE ( 'NONE', #9660, #13237, #8082, .T. ) ;
#17874=CARTESIAN_POINT ( 'NONE',  ( 49.39887009976201426, 113.4706157781613598, -46.83140348491149041 ) ) ;
#17879=CARTESIAN_POINT ( 'NONE',  ( -40.09630628311408884, 94.23964578315411700, 84.16448747414683851 ) ) ;
#17889=CARTESIAN_POINT ( 'NONE',  ( -34.79755969384669356, 125.3640259171584290, 248.0123345355920890 ) ) ;
#17900=ORIENTED_EDGE ( 'NONE', *, *, #3919, .T. ) ;
#17901=ORIENTED_EDGE ( 'NONE', *, *, #9779, .F. ) ;
#17904=FACE_OUTER_BOUND ( 'NONE', #20136, .T. ) ;
#17921=ADVANCED_FACE ( 'NONE', ( #15082 ), #8281, .F. ) ;
#17924=CARTESIAN_POINT ( 'NONE',  ( 50.65705442791912816, 111.6851564030456103, -48.02593606187189579 ) ) ;
#17928=CARTESIAN_POINT ( 'NONE',  ( 51.42455095033977130, 113.4816418249608034, -44.85744920025983618 ) ) ;
#17940=CARTESIAN_POINT ( 'NONE',  ( 42.02709154643847000, 106.9581013127162379, 70.53115534494513383 ) ) ;
#17948=VERTEX_POINT ( 'NONE', #22484 ) ;
#17949=DIRECTION ( 'NONE',  ( -0.009188991635466048358, 0.7031977391749438810, -0.7109349492407661675 ) ) ;
#17953=PLANE ( 'NONE',  #11593 ) ;
#17956=CARTESIAN_POINT ( 'NONE',  ( 47.42620204064805023, 94.99786382055523859, -44.70385809434849733 ) ) ;
#17962=AXIS2_PLACEMENT_3D ( 'NONE', #7334, #14380, #21231 ) ;
#17968=CARTESIAN_POINT ( 'NONE',  ( -52.22280431992486882, 111.8670818006853551, -46.76325931430218219 ) ) ;
#17979=EDGE_CURVE ( 'NONE', #1849, #13913, #13653, .T. ) ;
#17995=AXIS2_PLACEMENT_3D ( 'NONE', #21769, #16204, #14482 ) ;
#18018=VERTEX_POINT ( 'NONE', #3204 ) ;
#18031=CARTESIAN_POINT ( 'NONE',  ( -34.79044227946425849, 119.3672327899910073, 248.5629954604718534 ) ) ;
#18037=CARTESIAN_POINT ( 'NONE',  ( 64.99457118636310327, 170.0000000000000284, -0.8400692238017243296 ) ) ;
#18040=DIRECTION ( 'NONE',  ( 0.009088227368120579963, 0.7109943316365083810, 0.7031390079522398251 ) ) ;
#18042=ORIENTED_EDGE ( 'NONE', *, *, #7097, .F. ) ;
#18045=CARTESIAN_POINT ( 'NONE',  ( -40.54068192821626582, 96.15465585523027414, -41.57304724140053764 ) ) ;
#18048=DIRECTION ( 'NONE',  ( 0.9999164797902015955, 6.965998958219364448E-18, -0.01292414190464157182 ) ) ;
#18076=DIRECTION ( 'NONE',  ( -0.01292394549866739996, -0.005513023399721131770, -0.9999012842304692006 ) ) ;
#18080=CARTESIAN_POINT ( 'NONE',  ( -39.06289137140529988, 108.3156947416822362, 72.76082051835628306 ) ) ;
#18083=CARTESIAN_POINT ( 'NONE',  ( 40.27217859821899282, 105.8205586461024552, 91.88447881881737089 ) ) ;
#18085=EDGE_LOOP ( 'NONE', ( #16067, #9096, #6789, #2312, #11850, #6373, #7467, #7988 ) ) ;
#18095=VERTEX_POINT ( 'NONE', #10681 ) ;
#18099=CARTESIAN_POINT ( 'NONE',  ( -53.22343177146392179, 169.4762627770265340, -94.31856662285323978 ) ) ;
#18100=CARTESIAN_POINT ( 'NONE',  ( -37.17546262443868699, 94.47305566264986965, 83.89071743665799374 ) ) ;
#18107=B_SPLINE_CURVE_WITH_KNOTS ( 'NONE', 3,
 ( #3248, #13406, #22529, #20377, #13508, #15134, #3145, #11664, #6494, #9936, #20484, #16964, #1228, #10059, #10274, #17076 ),
 .UNSPECIFIED., .F., .F.,
 ( 4, 2, 2, 2, 2, 2, 2, 4 ),
 ( 1.962615573354718958E-17, 0.0003919156718472174578, 0.0007838313436944152916, 0.001175747015541613342, 0.001567662687388811068, 0.002351494031083169439, 0.002743409702930348516, 0.003135325374777527159 ),
 .UNSPECIFIED. ) ;
#18119=VECTOR ( 'NONE', #21975, 1000.000000000000000 ) ;
#18124=ORIENTED_EDGE ( 'NONE', *, *, #1441, .T. ) ;
#18133=CARTESIAN_POINT ( 'NONE',  ( 51.99565694909048830, 170.0000000000000284, -0.6720553790413839046 ) ) ;
#18137=DIRECTION ( 'NONE',  ( -7.125109674243555432E-05, 0.9999848031710253382, -0.005512562950850175003 ) ) ;
#18139=ORIENTED_EDGE ( 'NONE', *, *, #6136, .F. ) ;
#18151=CIRCLE ( 'NONE', #12290, 77.00000000000002842 ) ;
#18157=CARTESIAN_POINT ( 'NONE',  ( 41.21551227533764461, 121.7015652700166868, 248.5325502308119781 ) ) ;
#18168=CIRCLE ( 'NONE', #17074, 2.000000000000001332 ) ;
#18169=CARTESIAN_POINT ( 'NONE',  ( 41.69668515243814966, 107.1131874321777673, 70.67272545139887541 ) ) ;
#18180=DIRECTION ( 'NONE',  ( 0.006595249899610063603, 0.8599936914359664897, 0.5102620438256224578 ) ) ;
#18181=ORIENTED_EDGE ( 'NONE', *, *, #649, .F. ) ;
#18201=ORIENTED_EDGE ( 'NONE', *, *, #7471, .T. ) ;
#18204=CARTESIAN_POINT ( 'NONE',  ( 39.50219223099954746, 95.87258117927862600, -43.09091958258431987 ) ) ;
#18214=DIRECTION ( 'NONE',  ( 0.01292394549866739996, 0.005513023399721131770, 0.9999012842304692006 ) ) ;
#18216=EDGE_CURVE ( 'NONE', #17590, #2480, #22419, .T. ) ;
#18219=EDGE_LOOP ( 'NONE', ( #4720, #411, #9422, #473 ) ) ;
#18221=CARTESIAN_POINT ( 'NONE',  ( -29.40402206585521938, 189.4003865961453528, -108.4455932242574505 ) ) ;
#18223=DIRECTION ( 'NONE',  ( 0.006717398120142096217, -0.8543148575185137705, 0.5197124212346833083 ) ) ;
#18226=EDGE_CURVE ( 'NONE', #18970, #4876, #16909, .T. ) ;
#18235=DIRECTION ( 'NONE',  ( -0.9999164797902017066, -6.965998958219365988E-18, 0.01292414190464157356 ) ) ;
#18237=CARTESIAN_POINT ( 'NONE',  ( 64.99457118636310327, 170.0000000000000284, -0.8400692238017243296 ) ) ;
#18239=CARTESIAN_POINT ( 'NONE',  ( 49.46945221206134136, 189.4905266074825647, -93.11355607525817391 ) ) ;
#18258=EDGE_LOOP ( 'NONE', ( #8391, #12351, #20738, #5497 ) ) ;
#18264=AXIS2_PLACEMENT_3D ( 'NONE', #1507, #3327, #6664 ) ;
#18273=ORIENTED_EDGE ( 'NONE', *, *, #22205, .T. ) ;
#18275=CARTESIAN_POINT ( 'NONE',  ( -51.96998430978931083, 113.4377214578606186, -43.52080978029741232 ) ) ;
#18286=CARTESIAN_POINT ( 'NONE',  ( 48.56361546678319030, 189.3893605493459233, -111.4534788612804732 ) ) ;
#18287=CARTESIAN_POINT ( 'NONE',  ( 50.79326848830832120, 189.6011149706892525, -73.06981957049683274 ) ) ;
#18314=VECTOR ( 'NONE', #10764, 999.9999999999998863 ) ;
#18316=ORIENTED_EDGE ( 'NONE', *, *, #8774, .T. ) ;
#18317=CARTESIAN_POINT ( 'NONE',  ( 40.92831632140950404, 108.1243619184625828, 71.56358903111998870 ) ) ;
#18323=LINE ( 'NONE', #9608, #9295 ) ;
#18325=ORIENTED_EDGE ( 'NONE', *, *, #169, .T. ) ;
#18333=EDGE_CURVE ( 'NONE', #12374, #14615, #18691, .T. ) ;
#18351=DIRECTION ( 'NONE',  ( -0.9999164797902015955, -6.965998958219364448E-18, 0.01292414190464157182 ) ) ;
#18352=EDGE_CURVE ( 'NONE', #17283, #665, #14411, .T. ) ;
#18364=CARTESIAN_POINT ( 'NONE',  ( -38.85236994344747075, 97.01168560782741679, 84.15801439602003597 ) ) ;
#18366=CARTESIAN_POINT ( 'NONE',  ( -41.49766754275730563, 95.16167501252658667, -43.27024962841050382 ) ) ;
#18369=ORIENTED_EDGE ( 'NONE', *, *, #11484, .T. ) ;
#18373=CARTESIAN_POINT ( 'NONE',  ( 27.99766143412564290, 170.0000000000008242, -0.3618759733291194713 ) ) ;
#18376=AXIS2_PLACEMENT_3D ( 'NONE', #15119, #7749, #4284 ) ;
#18385=CARTESIAN_POINT ( 'NONE',  ( -52.02336739672247035, 111.7630282158269068, -46.72747482793098328 ) ) ;
#18400=CARTESIAN_POINT ( 'NONE',  ( 50.92554597170246211, 189.6011917897851617, -73.05759422026605421 ) ) ;
#18408=CIRCLE ( 'NONE', #20587, 95.00000000000001421 ) ;
#18416=ORIENTED_EDGE ( 'NONE', *, *, #8572, .T. ) ;
#18417=CARTESIAN_POINT ( 'NONE',  ( 51.07319921393753503, 94.45452722260040446, 82.70828171889813518 ) ) ;
#18423=VECTOR ( 'NONE', #13342, 999.9999999999998863 ) ;
#18428=EDGE_CURVE ( 'NONE', #22554, #850, #20239, .T. ) ;
#18430=DIRECTION ( 'NONE',  ( -0.01292394549866740169, -0.005513023399719847208, -0.9999012842304693116 ) ) ;
#18433=DIRECTION ( 'NONE',  ( -0.9999164797902015955, -6.965998958219364448E-18, 0.01292414190464157182 ) ) ;
#18436=CARTESIAN_POINT ( 'NONE',  ( 64.42259306105445660, 139.7551263635816952, -45.17031240767400391 ) ) ;
#18445=EDGE_LOOP ( 'NONE', ( #15321, #20847, #21846, #1681 ) ) ;
#18449=FACE_OUTER_BOUND ( 'NONE', #2915, .T. ) ;
#18458=AXIS2_PLACEMENT_3D ( 'NONE', #20399, #8131, #6064 ) ;
#18463=CARTESIAN_POINT ( 'NONE',  ( 49.00729593383175597, 189.4940257501801568, -92.47283438282913437 ) ) ;
#18464=VERTEX_POINT ( 'NONE', #20140 ) ;
#18468=ORIENTED_EDGE ( 'NONE', *, *, #7379, .F. ) ;
#18473=VERTEX_POINT ( 'NONE', #21855 ) ;
#18474=DIRECTION ( 'NONE',  ( 7.125109674161238737E-05, -0.9999848031710253382, 0.005512562950850163727 ) ) ;
#18477=EDGE_CURVE ( 'NONE', #444, #7056, #10727, .T. ) ;
#18478=EDGE_LOOP ( 'NONE', ( #3353, #12713, #15324, #5412, #9192, #2320, #10227, #13898 ) ) ;
#18480=ADVANCED_FACE ( 'NONE', ( #18449 ), #16402, .T. ) ;
#18499=AXIS2_PLACEMENT_3D ( 'NONE', #2871, #13236, #15722 ) ;
#18500=ORIENTED_EDGE ( 'NONE', *, *, #15700, .F. ) ;
#18502=LINE ( 'NONE', #823, #3628 ) ;
#18503=CARTESIAN_POINT ( 'NONE',  ( -50.76749586831994066, 109.7796205288052107, -46.01748440586237621 ) ) ;
#18507=CARTESIAN_POINT ( 'NONE',  ( -51.99565694909051672, 170.0000000000000284, 0.6720553790413400508 ) ) ;
#18522=EDGE_LOOP ( 'NONE', ( #15191, #15383, #14911, #18468, #12517 ) ) ;
#18524=CARTESIAN_POINT ( 'NONE',  ( -48.80449223365644684, 105.5072037373731888, 92.81729778463858338 ) ) ;
#18531=ORIENTED_EDGE ( 'NONE', *, *, #18352, .T. ) ;
#18535=DIRECTION ( 'NONE',  ( -0.9999164797902015955, -6.965998958219364448E-18, 0.01292414190464157182 ) ) ;
#18547=CARTESIAN_POINT ( 'NONE',  ( 66.07231611197045140, 94.48610424851698042, 82.54302267323384967 ) ) ;
#18552=VERTEX_POINT ( 'NONE', #11558 ) ;
#18560=CIRCLE ( 'NONE', #212, 87.00000000000001421 ) ;
#18565=CARTESIAN_POINT ( 'NONE',  ( -47.41909850602771570, 108.0982075334647163, 200.0025971627301260 ) ) ;
#18568=FACE_OUTER_BOUND ( 'NONE', #3091, .T. ) ;
#18570=CARTESIAN_POINT ( 'NONE',  ( 50.52662230413528732, 189.4876967392748384, -93.64056134612683024 ) ) ;
#18574=ORIENTED_EDGE ( 'NONE', *, *, #4292, .T. ) ;
#18592=CARTESIAN_POINT ( 'NONE',  ( -52.60896573992756942, 111.9218655255082382, -46.77848885693064318 ) ) ;
#18596=EDGE_CURVE ( 'NONE', #11284, #10697, #22305, .T. ) ;
#18606=DIRECTION ( 'NONE',  ( -0.9999164797902015955, -6.965998958219364448E-18, 0.01292414190464157182 ) ) ;
#18615=AXIS2_PLACEMENT_3D ( 'NONE', #13719, #18974, #3231 ) ;
#18616=EDGE_CURVE ( 'NONE', #2170, #4358, #19151, .T. ) ;
#18621=CARTESIAN_POINT ( 'NONE',  ( 49.05359984820991315, 95.50335886808198893, -45.57402858099457177 ) ) ;
#18622=DIRECTION ( 'NONE',  ( 0.9999164797902015955, 6.965998958219364448E-18, -0.01292414190464157182 ) ) ;
#18623=ORIENTED_EDGE ( 'NONE', *, *, #3526, .F. ) ;
#18633=CARTESIAN_POINT ( 'NONE',  ( 41.19638261157624015, 121.2962013336460956, 247.0525242307099347 ) ) ;
#18638=CARTESIAN_POINT ( 'NONE',  ( -52.18379134969580235, 189.4892127681350189, -92.03799725394125630 ) ) ;
#18647=CYLINDRICAL_SURFACE ( 'NONE', #3333, 87.00000000000001421 ) ;
#18649=DIRECTION ( 'NONE',  ( -0.01292394549866741904, -0.005513023399721091004, -0.9999012842304693116 ) ) ;
#18656=AXIS2_PLACEMENT_3D ( 'NONE', #4689, #6451, #13463 ) ;
#18664=CARTESIAN_POINT ( 'NONE',  ( 41.08943404267284905, 95.79007946549236863, 84.02896320188966683 ) ) ;
#18666=CARTESIAN_POINT ( 'NONE',  ( -39.06500206180663071, 108.1243619184625118, 72.59752038349127190 ) ) ;
#18668=EDGE_CURVE ( 'NONE', #1318, #8537, #14036, .T. ) ;
#18672=CARTESIAN_POINT ( 'NONE',  ( 14.14167086503323034, 113.6998737626107641, 126.9321988120954643 ) ) ;
#18690=CARTESIAN_POINT ( 'NONE',  ( -20.57109388430227881, 136.7551719540686008, -44.05520973278501629 ) ) ;
#18691=LINE ( 'NONE', #15285, #17696 ) ;
#18696=CARTESIAN_POINT ( 'NONE',  ( -52.60896573992756942, 111.9218655255082382, -46.77848885693064318 ) ) ;
#18698=CIRCLE ( 'NONE', #20166, 85.00000000000001421 ) ;
#18700=CARTESIAN_POINT ( 'NONE',  ( -16.77435518417359717, 141.3748088146942621, 249.6913015425559195 ) ) ;
#18703=VECTOR ( 'NONE', #12983, 999.9999999999998863 ) ;
#18707=CARTESIAN_POINT ( 'NONE',  ( -51.12349514068515077, 113.1361128394719771, -43.53008790071018552 ) ) ;
#18708=CARTESIAN_POINT ( 'NONE',  ( 23.22251776072470619, 138.3748544051812246, 249.1908735552227938 ) ) ;
#18709=CARTESIAN_POINT ( 'NONE',  ( -51.99565694909051672, 170.0000000000000284, 0.6720553790413400508 ) ) ;
#18716=ADVANCED_FACE ( 'NONE', ( #3598 ), #594, .T. ) ;
#18717=ORIENTED_EDGE ( 'NONE', *, *, #10497, .T. ) ;
#18731=CARTESIAN_POINT ( 'NONE',  ( 49.36348188940251447, 95.91501852516964277, -46.25422087729876353 ) ) ;
#18734=AXIS2_PLACEMENT_3D ( 'NONE', #21157, #19551, #262 ) ;
#18740=ADVANCED_FACE ( 'NONE', ( #20823 ), #15926, .T. ) ;
#18743=DIRECTION ( 'NONE',  ( 7.125109674161246868E-05, -0.9999848031710252272, 0.005512562950850154186 ) ) ;
#18756=AXIS2_PLACEMENT_3D ( 'NONE', #11860, #18622, #1406 ) ;
#18765=DIRECTION ( 'NONE',  ( 7.125109674161246868E-05, -0.9999848031710252272, 0.005512562950850154186 ) ) ;
#18771=DIRECTION ( 'NONE',  ( -0.01292394549866704608, -0.005513023399720698957, -0.9999012842304692006 ) ) ;
#18774=VECTOR ( 'NONE', #21316, 1000.000000000000114 ) ;
#18775=ADVANCED_FACE ( 'NONE', ( #20084 ), #1215, .T. ) ;
#18777=AXIS2_PLACEMENT_3D ( 'NONE', #18709, #9877, #22579 ) ;
#18783=CARTESIAN_POINT ( 'NONE',  ( -38.77137772201017185, 125.3750519639578727, 250.0638336716716310 ) ) ;
#18787=EDGE_CURVE ( 'NONE', #956, #2170, #12214, .T. ) ;
#18789=CARTESIAN_POINT ( 'NONE',  ( -48.91807906390275207, 94.48610424851698042, 84.02929899226762700 ) ) ;
#18793=AXIS2_PLACEMENT_3D ( 'NONE', #13950, #17633, #11156 ) ;
#18798=ORIENTED_EDGE ( 'NONE', *, *, #11782, .T. ) ;
#18803=ADVANCED_FACE ( 'NONE', ( #3434 ), #10336, .T. ) ;
#18806=DIRECTION ( 'NONE',  ( 7.125109674161246868E-05, -0.9999848031710252272, 0.005512562950850154186 ) ) ;
#18808=DIRECTION ( 'NONE',  ( 7.125109674161246868E-05, -0.9999848031710253382, 0.005512562950850155054 ) ) ;
#18814=CARTESIAN_POINT ( 'NONE',  ( 42.57010254367627766, 108.0286580773774148, 198.5854920750244901 ) ) ;
#18818=CYLINDRICAL_SURFACE ( 'NONE', #6619, 2.000000000000001332 ) ;
#18822=CARTESIAN_POINT ( 'NONE',  ( 42.57338467509045188, 108.0982075334647163, 198.8394243913123489 ) ) ;
#18824=EDGE_CURVE ( 'NONE', #8679, #11415, #10216, .T. ) ;
#18827=CIRCLE ( 'NONE', #14825, 93.00000000000001421 ) ;
#18830=ORIENTED_EDGE ( 'NONE', *, *, #18616, .F. ) ;
#18831=CARTESIAN_POINT ( 'NONE',  ( -50.63964423113515778, 108.5889086405974240, -43.51127046276314303 ) ) ;
#18835=AXIS2_PLACEMENT_3D ( 'NONE', #12217, #14172, #5394 ) ;
#18839=CARTESIAN_POINT ( 'NONE',  ( 51.57037466492827349, 109.8957517466449048, -44.83956295643738343 ) ) ;
#18843=DIRECTION ( 'NONE',  ( 0.9999164797902015955, 6.965998958219364448E-18, -0.01292414190464157182 ) ) ;
#18851=VECTOR ( 'NONE', #18606, 1000.000000000000000 ) ;
#18855=ORIENTED_EDGE ( 'NONE', *, *, #18477, .T. ) ;
#18863=CARTESIAN_POINT ( 'NONE',  ( -52.54463837782685687, 189.4882857640628799, -92.20149275433632852 ) ) ;
#18870=AXIS2_PLACEMENT_3D ( 'NONE', #16737, #759, #13166 ) ;
#18886=DIRECTION ( 'NONE',  ( 0.01292394549866740343, 0.005513023399721065851, 0.9999012842304692006 ) ) ;
#18890=DIRECTION ( 'NONE',  ( 0.9999164797902017066, 6.965998958219365988E-18, -0.01292414190464157356 ) ) ;
#18891=CARTESIAN_POINT ( 'NONE',  ( -51.60252166286891651, 189.5983001498699423, -72.25694281118451556 ) ) ;
#18894=EDGE_CURVE ( 'NONE', #726, #13165, #20881, .T. ) ;
#18923=EDGE_CURVE ( 'NONE', #17586, #1365, #5222, .T. ) ;
#18924=FACE_OUTER_BOUND ( 'NONE', #1355, .T. ) ;
#18928=DIRECTION ( 'NONE',  ( -7.125109674161246868E-05, 0.9999848031710253382, -0.005512562950850155054 ) ) ;
#18933=DIRECTION ( 'NONE',  ( -0.01292394549866737741, -0.005513023399721125699, -0.9999012842304693116 ) ) ;
#18941=CARTESIAN_POINT ( 'NONE',  ( 51.64825477779187679, 109.2957511350118409, -44.83726143016509269 ) ) ;
#18946=DIRECTION ( 'NONE',  ( 0.006837993415046672921, 0.8485676841065771248, 0.5290426517172845955 ) ) ;
#18952=EDGE_LOOP ( 'NONE', ( #17620, #22501, #14510, #19422 ) ) ;
#18953=CARTESIAN_POINT ( 'NONE',  ( 48.37538072690065150, 95.13735778864688086, -44.95265272237791976 ) ) ;
#18955=ORIENTED_EDGE ( 'NONE', *, *, #7267, .T. ) ;
#18959=ORIENTED_EDGE ( 'NONE', *, *, #19630, .T. ) ;
#18968=CARTESIAN_POINT ( 'NONE',  ( -51.58190103849386787, 189.4920902165459609, -91.52380460646458005 ) ) ;
#18970=VERTEX_POINT ( 'NONE', #3882 ) ;
#18974=DIRECTION ( 'NONE',  ( 0.006837993415046672921, 0.8485676841065771248, 0.5290426517172845955 ) ) ;
#18978=ORIENTED_EDGE ( 'NONE', *, *, #11027, .F. ) ;
#18987=CARTESIAN_POINT ( 'NONE',  ( -20.15201938634779921, 7.270595330592057870, -11.63220634452945390 ) ) ;
#19004=DIRECTION ( 'NONE',  ( -0.01292394549866739996, -0.005513023399721131770, -0.9999012842304692006 ) ) ;
#19021=CIRCLE ( 'NONE', #15029, 95.00000000000001421 ) ;
#19032=CARTESIAN_POINT ( 'NONE',  ( 39.33558597195864337, 105.5072037373731604, 91.67806775769213345 ) ) ;
#19035=AXIS2_PLACEMENT_3D ( 'NONE', #2380, #19924, #11106 ) ;
#19036=CYLINDRICAL_SURFACE ( 'NONE', #12818, 2.000000000000001332 ) ;
#19040=CARTESIAN_POINT ( 'NONE',  ( 21.01742933042251948, 97.26594046717957553, 78.58734125711376350 ) ) ;
#19041=EDGE_CURVE ( 'NONE', #309, #3054, #1940, .T. ) ;
#19043=CARTESIAN_POINT ( 'NONE',  ( -50.56656660976580753, 108.3817487785542397, -43.51107281728322107 ) ) ;
#19052=DIRECTION ( 'NONE',  ( -7.125109674161230605E-05, 0.9999848031710253382, -0.005512562950850140309 ) ) ;
#19056=CARTESIAN_POINT ( 'NONE',  ( 49.99582398951007889, 170.0000000000000284, -0.6462070952321007367 ) ) ;
#19058=B_SPLINE_CURVE_WITH_KNOTS ( 'NONE', 3,
 ( #12250, #4878, #1457, #10407, #17426, #13639, #15371, #10077, #8435, #22439 ),
 .UNSPECIFIED., .F., .F.,
 ( 4, 2, 2, 2, 4 ),
 ( -8.944271960021110598E-06, 0.0009933947872009813579, 0.001995733846361983505, 0.002998072905522986085, 0.004000411964683988665 ),
 .UNSPECIFIED. ) ;
#19074=EDGE_CURVE ( 'NONE', #552, #8312, #13694, .T. ) ;
#19077=CARTESIAN_POINT ( 'NONE',  ( 49.42284594772163331, 139.7551263635817236, -44.97643735496247785 ) ) ;
#19091=EDGE_CURVE ( 'NONE', #18552, #9134, #3404, .T. ) ;
#19093=AXIS2_PLACEMENT_3D ( 'NONE', #14414, #20928, #12681 ) ;
#19103=EDGE_CURVE ( 'NONE', #11611, #6360, #910, .T. ) ;
#19106=EDGE_CURVE ( 'NONE', #6085, #15577, #7807, .T. ) ;
#19132=AXIS2_PLACEMENT_3D ( 'NONE', #12416, #19403, #14029 ) ;
#19140=ORIENTED_EDGE ( 'NONE', *, *, #13196, .F. ) ;
#19146=CARTESIAN_POINT ( 'NONE',  ( 49.00068018611270304, 169.5754971982215125, -77.63860598097826937 ) ) ;
#19151=CIRCLE ( 'NONE', #82, 2.000000000000001332 ) ;
#19165=ORIENTED_EDGE ( 'NONE', *, *, #14926, .T. ) ;
#19167=LINE ( 'NONE', #117, #12898 ) ;
#19168=ORIENTED_EDGE ( 'NONE', *, *, #7695, .T. ) ;
#19169=CARTESIAN_POINT ( 'NONE',  ( 50.83832527469255780, 109.9515020747574852, -44.83040843917926566 ) ) ;
#19178=DIRECTION ( 'NONE',  ( -0.9999164797902015955, -6.965998958219364448E-18, 0.01292414190464157182 ) ) ;
#19185=ORIENTED_EDGE ( 'NONE', *, *, #15855, .F. ) ;
#19191=ORIENTED_EDGE ( 'NONE', *, *, #2807, .T. ) ;
#19192=EDGE_LOOP ( 'NONE', ( #19838, #6208 ) ) ;
#19195=VERTEX_POINT ( 'NONE', #9849 ) ;
#19197=DIRECTION ( 'NONE',  ( -0.9999164797902015955, -6.965998958219364448E-18, 0.01292414190464157182 ) ) ;
#19209=VERTEX_POINT ( 'NONE', #4215 ) ;
#19232=LINE ( 'NONE', #56, #4917 ) ;
#19240=CARTESIAN_POINT ( 'NONE',  ( -37.99233741293296163, 107.0009574002254453, 0.8384088582799177347 ) ) ;
#19241=EDGE_CURVE ( 'NONE', #16738, #19195, #7664, .T. ) ;
#19250=CARTESIAN_POINT ( 'NONE',  ( -40.54068192821626582, 96.15465585523027414, -41.57304724140053764 ) ) ;
#19252=DIRECTION ( 'NONE',  ( -0.01292394549866738261, -0.005513023399719314648, -0.9999012842304692006 ) ) ;
#19257=DIRECTION ( 'NONE',  ( 7.125109674161818785E-05, -0.9999848031710252272, 0.005512562950850596541 ) ) ;
#19266=DIRECTION ( 'NONE',  ( 7.125109674161246868E-05, -0.9999848031710252272, 0.005512562950850154186 ) ) ;
#19272=CARTESIAN_POINT ( 'NONE',  ( 50.89197640125190958, 108.0238286078847523, 68.68741454989820738 ) ) ;
#19273=CARTESIAN_POINT ( 'NONE',  ( 41.42315785391630811, 144.7550503794368524, -44.90060703447959156 ) ) ;
#19275=LINE ( 'NONE', #3539, #2231 ) ;
#19281=ORIENTED_EDGE ( 'NONE', *, *, #7734, .T. ) ;
#19286=CARTESIAN_POINT ( 'NONE',  ( 51.08127105622416053, 111.8896246953612206, -48.10680864709630100 ) ) ;
#19305=EDGE_CURVE ( 'NONE', #13285, #16331, #3403, .T. ) ;
#19317=CARTESIAN_POINT ( 'NONE',  ( -35.42010074854528767, 108.0982075334647163, 199.8475074598744357 ) ) ;
#19327=DIRECTION ( 'NONE',  ( 0.01246513159389315249, 0.2641402835564749529, 0.9644037178988122960 ) ) ;
#19330=ORIENTED_EDGE ( 'NONE', *, *, #15841, .F. ) ;
#19333=EDGE_LOOP ( 'NONE', ( #6507, #18574, #3873, #2063, #9839 ) ) ;
#19335=AXIS2_PLACEMENT_3D ( 'NONE', #8628, #11989, #12102 ) ;
#19355=ORIENTED_EDGE ( 'NONE', *, *, #17103, .F. ) ;
#19366=CARTESIAN_POINT ( 'NONE',  ( 51.58262974252190958, 107.1441749712451639, 69.90890102575978915 ) ) ;
#19370=VERTEX_POINT ( 'NONE', #8782 ) ;
#19374=CARTESIAN_POINT ( 'NONE',  ( -40.92987198850381958, 97.39926864640101201, 83.83894969480016357 ) ) ;
#19381=CARTESIAN_POINT ( 'NONE',  ( -10.91052170081621853, 113.6767190643319196, 123.0557169659435459 ) ) ;
#19387=DIRECTION ( 'NONE',  ( 0.01292394549867042185, 0.005513023399718316314, 0.9999012842304693116 ) ) ;
#19392=CARTESIAN_POINT ( 'NONE',  ( 49.56017638316297536, 109.8092428479078961, -47.32487478585164808 ) ) ;
#19394=EDGE_LOOP ( 'NONE', ( #8497, #19165, #19598, #18139 ) ) ;
#19395=CARTESIAN_POINT ( 'NONE',  ( -48.91844876508264406, 94.45452722259994971, 84.00069590936301722 ) ) ;
#19398=CARTESIAN_POINT ( 'NONE',  ( 51.42485355984464945, 109.2346207959984241, -44.83403687369097668 ) ) ;
#19403=DIRECTION ( 'NONE',  ( 0.9999164797902015955, 6.965998958219364448E-18, -0.01292414190464157182 ) ) ;
#19409=DIRECTION ( 'NONE',  ( -0.006837993415046672921, -0.8485676841065771248, -0.5290426517172845955 ) ) ;
#19415=CARTESIAN_POINT ( 'NONE',  ( -10.85624112972181621, 113.6998737626107641, 127.2553023597115214 ) ) ;
#19416=AXIS2_PLACEMENT_3D ( 'NONE', #6600, #16973, #5295 ) ;
#19417=EDGE_CURVE ( 'NONE', #726, #22603, #8547, .T. ) ;
#19421=FACE_OUTER_BOUND ( 'NONE', #14517, .T. ) ;
#19422=ORIENTED_EDGE ( 'NONE', *, *, #710, .F. ) ;
#19427=CARTESIAN_POINT ( 'NONE',  ( -10.85795115604361349, 137.6995090387153482, 127.1230008488911096 ) ) ;
#19447=CARTESIAN_POINT ( 'NONE',  ( 40.87255160414490973, 95.04007462656775829, -44.54585608918304729 ) ) ;
#19449=ADVANCED_FACE ( 'NONE', ( #3956 ), #1236, .F. ) ;
#19451=CARTESIAN_POINT ( 'NONE',  ( -40.80932907711049751, 95.23503300788487991, 83.16719596654198199 ) ) ;
#19457=VECTOR ( 'NONE', #3179, 1000.000000000000000 ) ;
#19458=DIRECTION ( 'NONE',  ( 7.125109674161246868E-05, -0.9999848031710253382, 0.005512562950850155054 ) ) ;
#19459=TOROIDAL_SURFACE ( 'NONE', #9187, 85.00000000000000000, 2.000000000000000000 ) ;
#19463=DIRECTION ( 'NONE',  ( -0.01292394549866740169, -0.005513023399721131770, -0.9999012842304693116 ) ) ;
#19464=ORIENTED_EDGE ( 'NONE', *, *, #20826, .F. ) ;
#19469=CARTESIAN_POINT ( 'NONE',  ( -63.91682626075579066, 94.48610424851698042, 84.22316112083727546 ) ) ;
#19482=ADVANCED_BREP_SHAPE_REPRESENTATION ( '', ( #9632, #6292 ), #7747 ) ;
#19484=DIRECTION ( 'NONE',  ( 0.006717398120142096217, -0.8543148575185137705, 0.5197124212346833083 ) ) ;
#19487=CIRCLE ( 'NONE', #15491, 1.999999999999998446 ) ;
#19489=FACE_OUTER_BOUND ( 'NONE', #5865, .T. ) ;
#19494=FACE_OUTER_BOUND ( 'NONE', #17169, .T. ) ;
#19509=VERTEX_POINT ( 'NONE', #21969 ) ;
#19511=CARTESIAN_POINT ( 'NONE',  ( 14.19424140980583537, 137.7226637369942068, 130.9994826950430422 ) ) ;
#19513=CARTESIAN_POINT ( 'NONE',  ( -49.63640462543862242, 95.17726600392212788, -43.75321583467091813 ) ) ;
#19514=AXIS2_PLACEMENT_3D ( 'NONE', #9802, #4500, #8061 ) ;
#19522=B_SPLINE_CURVE_WITH_KNOTS ( 'NONE', 3,
 ( #22510, #20585, #20364, #2908, #1650, #9919, #17272, #16944 ),
 .UNSPECIFIED., .F., .F.,
 ( 4, 2, 2, 4 ),
 ( 6.938893903907228378E-18, 0.0005562605569428313076, 0.001112521113885655676, 0.002225042227771339108 ),
 .UNSPECIFIED. ) ;
#19523=VECTOR ( 'NONE', #17119, 999.9999999999998863 ) ;
#19529=ORIENTED_EDGE ( 'NONE', *, *, #14846, .T. ) ;
#19539=AXIS2_PLACEMENT_3D ( 'NONE', #2740, #6176, #9751 ) ;
#19542=DIRECTION ( 'NONE',  ( -0.01292394549866744159, -0.005513023399721241925, -0.9999012842304693116 ) ) ;
#19544=CARTESIAN_POINT ( 'NONE',  ( 48.56361546678319030, 189.3893605493459233, -111.4534788612804732 ) ) ;
#19545=ORIENTED_EDGE ( 'NONE', *, *, #8003, .T. ) ;
#19551=DIRECTION ( 'NONE',  ( -7.125109674161259066E-05, 0.9999848031710252272, -0.005512562950850163727 ) ) ;
#19555=ORIENTED_EDGE ( 'NONE', *, *, #1116, .F. ) ;
#19561=CARTESIAN_POINT ( 'NONE',  ( -15.05589034484066246, 113.6998737626107641, 127.3095837557110315 ) ) ;
#19581=AXIS2_PLACEMENT_3D ( 'NONE', #18133, #11110, #5797 ) ;
#19594=DIRECTION ( 'NONE',  ( -0.9999164797902017066, -6.965998958219367529E-18, 0.01292414190464157182 ) ) ;
#19598=ORIENTED_EDGE ( 'NONE', *, *, #15459, .T. ) ;
#19604=EDGE_CURVE ( 'NONE', #6519, #8189, #12825, .T. ) ;
#19607=EDGE_CURVE ( 'NONE', #2673, #16738, #18323, .T. ) ;
#19610=CARTESIAN_POINT ( 'NONE',  ( 53.19480552330409751, 129.3639651298425406, 246.8529597961802438 ) ) ;
#19618=EDGE_CURVE ( 'NONE', #8537, #19370, #19922, .T. ) ;
#19624=VECTOR ( 'NONE', #11147, 1000.000000000000114 ) ;
#19630=EDGE_CURVE ( 'NONE', #9213, #15636, #2479, .T. ) ;
#19636=VERTEX_POINT ( 'NONE', #3382 ) ;
#19638=CARTESIAN_POINT ( 'NONE',  ( 65.91132412060191825, 106.8061942917681790, 70.08737598725748796 ) ) ;
#19641=CARTESIAN_POINT ( 'NONE',  ( 51.05126519560737108, 95.51270090492249665, 81.01128809578769108 ) ) ;
#19643=ORIENTED_EDGE ( 'NONE', *, *, #13488, .T. ) ;
#19649=PLANE ( 'NONE',  #21528 ) ;
#19653=DIRECTION ( 'NONE',  ( -0.9999164797902017066, -6.965998958219367529E-18, 0.01292414190464157182 ) ) ;
#19662=ORIENTED_EDGE ( 'NONE', *, *, #20826, .T. ) ;
#19677=EDGE_LOOP ( 'NONE', ( #889, #4654, #6309, #12350 ) ) ;
#19682=CARTESIAN_POINT ( 'NONE',  ( 63.56236266363622889, 189.3893605493459233, -111.6473409898501075 ) ) ;
#19684=CARTESIAN_POINT ( 'NONE',  ( 14.14224087380716455, 105.6999953372425409, 126.9762993157022777 ) ) ;
#19693=VECTOR ( 'NONE', #11353, 999.9999999999998863 ) ;
#19700=DIRECTION ( 'NONE',  ( 0.01292394549866743465, 0.005513023399721021615, 0.9999012842304692006 ) ) ;
#19703=EDGE_LOOP ( 'NONE', ( #9648, #7628, #15557, #12255, #4430, #9086, #17321, #499 ) ) ;
#19704=DIRECTION ( 'NONE',  ( 0.9999164797902015955, 6.965998958219364448E-18, -0.01292414190464157182 ) ) ;
#19706=ORIENTED_EDGE ( 'NONE', *, *, #16286, .F. ) ;
#19709=ADVANCED_FACE ( 'NONE', ( #17295 ), #17375, .F. ) ;
#19725=AXIS2_PLACEMENT_3D ( 'NONE', #22304, #13620, #4861 ) ;
#19729=ADVANCED_FACE ( 'NONE', ( #22307 ), #13625, .F. ) ;
#19737=AXIS2_PLACEMENT_3D ( 'NONE', #8993, #14079, #7384 ) ;
#19761=CARTESIAN_POINT ( 'NONE',  ( 41.15884018182899950, 107.0346074789500506, 92.70501406802365807 ) ) ;
#19767=EDGE_CURVE ( 'NONE', #14285, #15416, #16970, .T. ) ;
#19772=CARTESIAN_POINT ( 'NONE',  ( 39.67545195212834130, 95.60340224533959486, -43.55612573487053396 ) ) ;
#19777=CARTESIAN_POINT ( 'NONE',  ( -66.44851505496320954, 169.3797848675314128, -111.6488252521261160 ) ) ;
#19788=ORIENTED_EDGE ( 'NONE', *, *, #16389, .F. ) ;
#19790=FACE_OUTER_BOUND ( 'NONE', #8212, .T. ) ;
#19798=TOROIDAL_SURFACE ( 'NONE', #21287, 4.000000000000000000, 2.000000000000000000 ) ;
#19799=ORIENTED_EDGE ( 'NONE', *, *, #11027, .T. ) ;
#19801=DIRECTION ( 'NONE',  ( 0.9999164797902015955, 6.965998958219364448E-18, -0.01292414190464157182 ) ) ;
#19802=CARTESIAN_POINT ( 'NONE',  ( -41.08973838174756565, 106.8061942917681790, 71.47038841247318430 ) ) ;
#19804=CARTESIAN_POINT ( 'NONE',  ( -47.41895600383423215, 106.0982379271226677, 200.0136222886318365 ) ) ;
#19830=DIRECTION ( 'NONE',  ( 0.9999164797902015955, 6.965998958219364448E-18, -0.01292414190464157182 ) ) ;
#19833=CYLINDRICAL_SURFACE ( 'NONE', #639, 7.921742784567035400 ) ;
#19838=ORIENTED_EDGE ( 'NONE', *, *, #8715, .T. ) ;
#19841=CARTESIAN_POINT ( 'NONE',  ( -41.00454908889594918, 95.41939025383068440, -42.83076017402247260 ) ) ;
#19845=CARTESIAN_POINT ( 'NONE',  ( 64.42478219708148401, 94.99786382055523859, -44.92356850672740620 ) ) ;
#19851=VECTOR ( 'NONE', #1762, 1000.000000000000000 ) ;
#19863=DIRECTION ( 'NONE',  ( -0.01292394549866737220, -0.005513023399725441691, -0.9999012842304692006 ) ) ;
#19864=LINE ( 'NONE', #11043, #21415 ) ;
#19866=ORIENTED_EDGE ( 'NONE', *, *, #7447, .F. ) ;
#19870=EDGE_CURVE ( 'NONE', #11611, #11415, #5207, .T. ) ;
#19881=CARTESIAN_POINT ( 'NONE',  ( 41.20572975695933593, 107.5148010522800064, 93.02654324256212703 ) ) ;
#19890=ADVANCED_FACE ( 'NONE', ( #8998 ), #5736, .F. ) ;
#19901=DIRECTION ( 'NONE',  ( 7.125109674143708543E-05, -0.9999848031710252272, 0.005512562950848880899 ) ) ;
#19904=DIRECTION ( 'NONE',  ( 7.125109674143708543E-05, -0.9999848031710252272, 0.005512562950848880899 ) ) ;
#19912=ORIENTED_EDGE ( 'NONE', *, *, #12170, .F. ) ;
#19915=CARTESIAN_POINT ( 'NONE',  ( 42.65965783573783909, 106.8159614793892018, 70.39661456005998730 ) ) ;
#19917=CIRCLE ( 'NONE', #149, 93.00000000000001421 ) ;
#19920=CIRCLE ( 'NONE', #21747, 2.000000000000001332 ) ;
#19922=LINE ( 'NONE', #4191, #5979 ) ;
#19924=DIRECTION ( 'NONE',  ( 0.9999164797902015955, 6.965998958219364448E-18, -0.01292414190464157182 ) ) ;
#19936=CARTESIAN_POINT ( 'NONE',  ( 50.79397376011281295, 189.4876967392748384, -93.64401692289283119 ) ) ;
#19945=DIRECTION ( 'NONE',  ( 0.9999164797902015955, 6.965998958219364448E-18, -0.01292414190464157182 ) ) ;
#19959=ORIENTED_EDGE ( 'NONE', *, *, #451, .F. ) ;
#19963=ORIENTED_EDGE ( 'NONE', *, *, #10767, .F. ) ;
#19974=CARTESIAN_POINT ( 'NONE',  ( -51.29282874781860357, 111.0349699797280181, -46.46914343950034265 ) ) ;
#19977=LINE ( 'NONE', #13456, #20985 ) ;
#19990=CARTESIAN_POINT ( 'NONE',  ( -38.81891740251079170, 107.5014370005211504, 91.63662627299856922 ) ) ;
#19992=PLANE ( 'NONE',  #12962 ) ;
#19993=PRESENTATION_STYLE_ASSIGNMENT (( #1993 ) ) ;
#19998=AXIS2_PLACEMENT_3D ( 'NONE', #3355, #5292, #13820 ) ;
#20006=EDGE_CURVE ( 'NONE', #22043, #17825, #22313, .T. ) ;
#20007=DIRECTION ( 'NONE',  ( 7.125109674161246868E-05, -0.9999848031710252272, 0.005512562950850154186 ) ) ;
#20012=ORIENTED_EDGE ( 'NONE', *, *, #2050, .F. ) ;
#20017=CARTESIAN_POINT ( 'NONE',  ( -50.59241450076314806, 108.3707227317548529, -45.51087538574414992 ) ) ;
#20026=DIRECTION ( 'NONE',  ( 0.01292394549866740169, 0.005513023399721125699, 0.9999012842304692006 ) ) ;
#20032=CARTESIAN_POINT ( 'NONE',  ( -25.02778843067846637, 55.00725983767637217, -132.4644698413844424 ) ) ;
#20036=CARTESIAN_POINT ( 'NONE',  ( -64.99457118636313169, 170.0000000000000284, 0.8400692238016805868 ) ) ;
#20045=CARTESIAN_POINT ( 'NONE',  ( -39.06279898716250187, 108.3240682923980245, 72.76796811295301382 ) ) ;
#20051=CARTESIAN_POINT ( 'NONE',  ( 49.78441085332420357, 189.4892230880255397, -93.35408680624050248 ) ) ;
#20052=DIRECTION ( 'NONE',  ( 0.01292394549866743812, 0.005513023399720639109, 0.9999012842304693116 ) ) ;
#20055=ORIENTED_EDGE ( 'NONE', *, *, #19630, .F. ) ;
#20056=ORIENTED_EDGE ( 'NONE', *, *, #11788, .F. ) ;
#20057=DIRECTION ( 'NONE',  ( -0.9999164797902015955, -6.965998958219364448E-18, 0.01292414190464157182 ) ) ;
#20061=CARTESIAN_POINT ( 'NONE',  ( -46.77041971896417749, 121.3072273804455250, 250.1896512867793945 ) ) ;
#20067=CARTESIAN_POINT ( 'NONE',  ( 20.96603472858061679, 99.74539563421257071, 74.61103786048234099 ) ) ;
#20070=CARTESIAN_POINT ( 'NONE',  ( -38.91889996795050166, 97.30032992285177329, 83.90116378639756078 ) ) ;
#20071=CARTESIAN_POINT ( 'NONE',  ( -46.79669995352260514, 127.3639955235004777, 248.1563991125460973 ) ) ;
#20080=ADVANCED_FACE ( 'NONE', ( #19421 ), #17497, .T. ) ;
#20082=ORIENTED_EDGE ( 'NONE', *, *, #20194, .F. ) ;
#20083=ORIENTED_EDGE ( 'NONE', *, *, #5677, .T. ) ;
#20084=FACE_OUTER_BOUND ( 'NONE', #5879, .T. ) ;
#20097=CARTESIAN_POINT ( 'NONE',  ( 9.942021649914385861, 113.6998737626107641, 126.9864802080949744 ) ) ;
#20099=DIRECTION ( 'NONE',  ( -0.009188991635466050092, 0.7031977391749439921, -0.7109349492407662785 ) ) ;
#20116=LINE ( 'NONE', #19777, #384 ) ;
#20130=ORIENTED_EDGE ( 'NONE', *, *, #15700, .T. ) ;
#20133=ORIENTED_EDGE ( 'NONE', *, *, #22183, .F. ) ;
#20136=EDGE_LOOP ( 'NONE', ( #12794, #18531, #21494, #5794, #1268, #21961, #17845 ) ) ;
#20140=CARTESIAN_POINT ( 'NONE',  ( 23.22230400743448442, 141.3748088146942621, 249.1743358663702566 ) ) ;
#20166=AXIS2_PLACEMENT_3D ( 'NONE', #4051, #12930, #11078 ) ;
#20179=DIRECTION ( 'NONE',  ( -0.01096700916508646859, 0.5290868411612599242, -0.8484968115555724388 ) ) ;
#20180=DIRECTION ( 'NONE',  ( -0.01246513159389404414, -0.2641402835564772844, -0.9644037178988117409 ) ) ;
#20187=AXIS2_PLACEMENT_3D ( 'NONE', #12405, #12300, #17578 ) ;
#20194=EDGE_CURVE ( 'NONE', #14615, #3864, #21248, .T. ) ;
#20211=CIRCLE ( 'NONE', #2622, 112.5000000000007105 ) ;
#20212=ORIENTED_EDGE ( 'NONE', *, *, #7951, .F. ) ;
#20221=ADVANCED_FACE ( 'NONE', ( #22610, #12433, #20917 ), #5175, .F. ) ;
#20239=CIRCLE ( 'NONE', #446, 3.399999999999985700 ) ;
#20243=CARTESIAN_POINT ( 'NONE',  ( -36.89904403399447119, 94.47498387040556622, 83.88519491590665211 ) ) ;
#20246=LINE ( 'NONE', #17155, #11895 ) ;
#20250=CARTESIAN_POINT ( 'NONE',  ( -49.07907105527128522, 106.8061942917681790, 71.57365230629126529 ) ) ;
#20251=ORIENTED_EDGE ( 'NONE', *, *, #11782, .F. ) ;
#20252=CIRCLE ( 'NONE', #19514, 4.199999999999997513 ) ;
#20253=APPLICATION_CONTEXT ( 'automotive_design' ) ;
#20254=CARTESIAN_POINT ( 'NONE',  ( 43.08423624159371457, 94.48610424851698042, 82.84014869562156491 ) ) ;
#20260=ORIENTED_EDGE ( 'NONE', *, *, #18923, .F. ) ;
#20268=DIRECTION ( 'NONE',  ( 0.9999164797902017066, 6.965998958219365988E-18, -0.01292414190464157356 ) ) ;
#20275=CARTESIAN_POINT ( 'NONE',  ( -39.47524343981440609, 107.3883277703368861, 71.96416890068093153 ) ) ;
#20281=ORIENTED_EDGE ( 'NONE', *, *, #21416, .T. ) ;
#20285=VECTOR ( 'NONE', #8268, 999.9999999999998863 ) ;
#20286=ORIENTED_EDGE ( 'NONE', *, *, #21950, .T. ) ;
#20288=AXIS2_PLACEMENT_3D ( 'NONE', #11753, #13262, #16821 ) ;
#20293=EDGE_CURVE ( 'NONE', #12189, #850, #19864, .T. ) ;
#20302=CARTESIAN_POINT ( 'NONE',  ( -48.91844876508264406, 94.45452722259994971, 84.00069590936301722 ) ) ;
#20318=DIRECTION ( 'NONE',  ( 0.9999164797902015955, 6.965998958219364448E-18, -0.01292414190464157182 ) ) ;
#20323=CARTESIAN_POINT ( 'NONE',  ( -50.99154849761720243, 113.0663986884224812, -43.53140896659793668 ) ) ;
#20327=CARTESIAN_POINT ( 'NONE',  ( -10.85567112094788200, 105.6999953372425409, 127.2994028633183063 ) ) ;
#20330=DIRECTION ( 'NONE',  ( 0.9999164797902015955, 6.965998958219364448E-18, -0.01292414190464157182 ) ) ;
#20331=LINE ( 'NONE', #6207, #18851 ) ;
#20337=AXIS2_PLACEMENT_3D ( 'NONE', #18373, #6851, #22559 ) ;
#20339=CARTESIAN_POINT ( 'NONE',  ( -49.99582398951010731, 170.0000000000000284, 0.6462070952320568828 ) ) ;
#20351=AXIS2_PLACEMENT_3D ( 'NONE', #7370, #16137, #375 ) ;
#20354=CARTESIAN_POINT ( 'NONE',  ( -37.48841359254407735, 105.6219042656103255, 92.61087584162487474 ) ) ;
#20361=DIRECTION ( 'NONE',  ( -0.01292394549866695240, -0.005513023399725255208, -0.9999012842304693116 ) ) ;
#20364=CARTESIAN_POINT ( 'NONE',  ( -40.51791796528902267, 94.71334217791753929, 83.69094846550264322 ) ) ;
#20374=CARTESIAN_POINT ( 'NONE',  ( 42.79028061014420103, 106.8061942917681364, 70.38622059413428644 ) ) ;
#20375=VERTEX_POINT ( 'NONE', #4017 ) ;
#20377=CARTESIAN_POINT ( 'NONE',  ( -49.15619943964080818, 107.7496120479954982, 70.42164486253489031 ) ) ;
#20381=DIRECTION ( 'NONE',  ( 7.125109674141484573E-05, -0.9999848031710252272, 0.005512562950851785694 ) ) ;
#20397=EDGE_CURVE ( 'NONE', #8988, #13237, #2772, .T. ) ;
#20398=CARTESIAN_POINT ( 'NONE',  ( -29.30063050186588214, 189.4444907833431273, -100.4463829504137209 ) ) ;
#20399=CARTESIAN_POINT ( 'NONE',  ( -10.85624112972181621, 113.6998737626107641, 127.2553023597115214 ) ) ;
#20409=EDGE_CURVE ( 'NONE', #13676, #11611, #20331, .T. ) ;
#20410=CYLINDRICAL_SURFACE ( 'NONE', #16375, 75.00000000000002842 ) ;
#20420=ADVANCED_FACE ( 'NONE', ( #10534 ), #17442, .F. ) ;
#20426=CARTESIAN_POINT ( 'NONE',  ( -20.57109388430227881, 136.7551719540686008, -44.05520973278501629 ) ) ;
#20434=CARTESIAN_POINT ( 'NONE',  ( 39.99665919160806027, 170.0000000000000284, -0.5169656761856848970 ) ) ;
#20438=CARTESIAN_POINT ( 'NONE',  ( 51.99565694909048830, 170.0000000000000284, -0.6720553790413839046 ) ) ;
#20443=CARTESIAN_POINT ( 'NONE',  ( 63.79288799738544213, 189.4876967392748384, -93.81203076765316951 ) ) ;
#20446=CARTESIAN_POINT ( 'NONE',  ( 47.71445816105992321, 95.00723670396115494, -44.72354054884888086 ) ) ;
#20453=ADVANCED_FACE ( 'NONE', ( #8672 ), #21065, .F. ) ;
#20464=VERTEX_POINT ( 'NONE', #12148 ) ;
#20465=DIRECTION ( 'NONE',  ( 0.01292394549866737741, 0.005513023399721125699, 0.9999012842304693116 ) ) ;
#20468=CARTESIAN_POINT ( 'NONE',  ( 14.14224087380716455, 105.6999953372425409, 126.9762993157022777 ) ) ;
#20471=DIRECTION ( 'NONE',  ( 0.01292394549866743465, 0.005513023399721021615, 0.9999012842304692006 ) ) ;
#20473=EDGE_CURVE ( 'NONE', #9134, #10176, #6406, .T. ) ;
#20477=EDGE_LOOP ( 'NONE', ( #12279, #2513 ) ) ;
#20482=ORIENTED_EDGE ( 'NONE', *, *, #3762, .F. ) ;
#20484=CARTESIAN_POINT ( 'NONE',  ( -50.07072918920412263, 106.9825899289013762, 71.40280719653912911 ) ) ;
#20492=CARTESIAN_POINT ( 'NONE',  ( -51.91681395539769994, 189.5996271088964704, -72.01216872995293272 ) ) ;
#20497=ORIENTED_EDGE ( 'NONE', *, *, #9480, .F. ) ;
#20502=CIRCLE ( 'NONE', #5084, 85.00000000000001421 ) ;
#20504=ORIENTED_EDGE ( 'NONE', *, *, #12315, .T. ) ;
#20511=AXIS2_PLACEMENT_3D ( 'NONE', #18783, #4978, #20381 ) ;
#20514=VECTOR ( 'NONE', #19704, 1000.000000000000000 ) ;
#20518=CARTESIAN_POINT ( 'NONE',  ( -38.41810471662249427, 96.40874508186763592, 84.69213597070189792 ) ) ;
#20529=DIRECTION ( 'NONE',  ( 0.01292394549866695240, 0.005513023399704438526, 0.9999012842304693116 ) ) ;
#20533=ORIENTED_EDGE ( 'NONE', *, *, #7532, .T. ) ;
#20542=AXIS2_PLACEMENT_3D ( 'NONE', #5014, #19266, #15509 ) ;
#20545=CARTESIAN_POINT ( 'NONE',  ( 49.39733347012933251, 108.7803151467795004, -46.95028962098039216 ) ) ;
#20549=DIRECTION ( 'NONE',  ( -0.01292394549866739996, -0.005513023399721131770, -0.9999012842304692006 ) ) ;
#20551=EDGE_CURVE ( 'NONE', #13286, #12735, #6848, .T. ) ;
#20555=EDGE_CURVE ( 'NONE', #22603, #726, #12278, .T. ) ;
#20570=ADVANCED_FACE ( 'NONE', ( #21201 ), #6019, .F. ) ;
#20578=VERTEX_POINT ( 'NONE', #21313 ) ;
#20579=EDGE_CURVE ( 'NONE', #14056, #16531, #3960, .T. ) ;
#20584=DIRECTION ( 'NONE',  ( 0.01246513159388064687, 0.2641402835564749529, 0.9644037178988124071 ) ) ;
#20585=CARTESIAN_POINT ( 'NONE',  ( -40.43031930919660510, 94.59775782198136085, 83.80669187395014319 ) ) ;
#20587=AXIS2_PLACEMENT_3D ( 'NONE', #21596, #16478, #498 ) ;
#20599=CARTESIAN_POINT ( 'NONE',  ( -21.36186403949424673, 189.4186551486401413, -105.2356049757943310 ) ) ;
#20613=CYLINDRICAL_SURFACE ( 'NONE', #5235, 112.5000000000000142 ) ;
#20618=CARTESIAN_POINT ( 'NONE',  ( -40.56069593696665976, 106.8539497625728103, 71.50607459554618117 ) ) ;
#20622=CIRCLE ( 'NONE', #17718, 95.00000000000001421 ) ;
#20636=CARTESIAN_POINT ( 'NONE',  ( 40.25303659951292445, 125.7553391191873544, -44.78072676432201860 ) ) ;
#20641=ORIENTED_EDGE ( 'NONE', *, *, #18428, .F. ) ;
#20644=CARTESIAN_POINT ( 'NONE',  ( -45.98860230557422568, 168.0766615966952884, -76.19549020176363285 ) ) ;
#20669=CARTESIAN_POINT ( 'NONE',  ( 49.22891015931647019, 112.6462081887176367, -44.82446383698096071 ) ) ;
#20678=VECTOR ( 'NONE', #17741, 1000.000000000000000 ) ;
#20680=VERTEX_POINT ( 'NONE', #2256 ) ;
#20681=CARTESIAN_POINT ( 'NONE',  ( 49.40009966013455056, 96.21415597129798414, -46.73627471826173974 ) ) ;
#20686=DIRECTION ( 'NONE',  ( 0.01096700916508646859, -0.5290868411612599242, 0.8484968115555724388 ) ) ;
#20691=DIRECTION ( 'NONE',  ( 7.125109674161246868E-05, -0.9999848031710253382, 0.005512562950850155054 ) ) ;
#20702=DIRECTION ( 'NONE',  ( -0.01292394549866739996, -0.005513023399721564584, -0.9999012842304692006 ) ) ;
#20703=AXIS2_PLACEMENT_3D ( 'NONE', #6050, #13080, #2603 ) ;
#20714=EDGE_LOOP ( 'NONE', ( #14827, #1454, #21954, #11798 ) ) ;
#20715=( GEOMETRIC_REPRESENTATION_CONTEXT ( 3 ) GLOBAL_UNCERTAINTY_ASSIGNED_CONTEXT ( ( #3489 ) ) GLOBAL_UNIT_ASSIGNED_CONTEXT ( ( #4259, #7602, #21709 ) ) REPRESENTATION_CONTEXT ( 'NONE', 'WORKASPACE' ) );
#20719=VERTEX_POINT ( 'NONE', #16069 ) ;
#20725=EDGE_CURVE ( 'NONE', #13213, #8991, #6948, .T. ) ;
#20737=LINE ( 'NONE', #12131, #1875 ) ;
#20738=ORIENTED_EDGE ( 'NONE', *, *, #10359, .F. ) ;
#20745=DIRECTION ( 'NONE',  ( 0.000000000000000000, -0.005512562964840580192, -0.9999848057093461140 ) ) ;
#20763=DIRECTION ( 'NONE',  ( 0.9999164797902015955, 6.965998958219364448E-18, -0.01292414190464157182 ) ) ;
#20770=CARTESIAN_POINT ( 'NONE',  ( -21.32529163372091219, 169.4339520569534159, -102.4060669292324661 ) ) ;
#20773=VERTEX_POINT ( 'NONE', #11674 ) ;
#20778=CARTESIAN_POINT ( 'NONE',  ( 50.35954681524507492, 109.7098288542535016, -44.82288763992134761 ) ) ;
#20787=VERTEX_POINT ( 'NONE', #9375 ) ;
#20788=CARTESIAN_POINT ( 'NONE',  ( 48.12222853284146140, 95.06897948779807450, -44.83367642559105803 ) ) ;
#20791=ORIENTED_EDGE ( 'NONE', *, *, #2780, .F. ) ;
#20820=DIRECTION ( 'NONE',  ( 0.9999164797902017066, 6.965998958219365988E-18, -0.01292414190464157356 ) ) ;
#20823=FACE_OUTER_BOUND ( 'NONE', #8288, .T. ) ;
#20826=EDGE_CURVE ( 'NONE', #21984, #16088, #13034, .T. ) ;
#20847=ORIENTED_EDGE ( 'NONE', *, *, #19074, .F. ) ;
#20856=DIRECTION ( 'NONE',  ( 0.9999164797902015955, 6.965998958219364448E-18, -0.01292414190464157182 ) ) ;
#20868=DIRECTION ( 'NONE',  ( 0.01292394549866739996, 0.005513023399720822122, 0.9999012842304692006 ) ) ;
#20881=LINE ( 'NONE', #15742, #19523 ) ;
#20885=EDGE_LOOP ( 'NONE', ( #3081, #19355, #15917, #4184 ) ) ;
#20886=ORIENTED_EDGE ( 'NONE', *, *, #20293, .T. ) ;
#20891=CARTESIAN_POINT ( 'NONE',  ( 51.23232595389467292, 111.9218655262938995, -48.12066054576542484 ) ) ;
#20893=CARTESIAN_POINT ( 'NONE',  ( 44.03004128744986190, 171.4878726268958360, -75.33468125154308836 ) ) ;
#20905=ORIENTED_EDGE ( 'NONE', *, *, #19607, .F. ) ;
#20908=CARTESIAN_POINT ( 'NONE',  ( -19.03062446302745414, 99.74539563421257071, 75.12800353666800390 ) ) ;
#20912=CYLINDRICAL_SURFACE ( 'NONE', #10721, 2.000000000000001332 ) ;
#20917=FACE_OUTER_BOUND ( 'NONE', #15915, .T. ) ;
#20919=EDGE_CURVE ( 'NONE', #12549, #19209, #21712, .T. ) ;
#20928=DIRECTION ( 'NONE',  ( 7.125109674161259066E-05, -0.9999848031710252272, 0.005512562950850163727 ) ) ;
#20930=VECTOR ( 'NONE', #1652, 1000.000000000000000 ) ;
#20934=LINE ( 'NONE', #10500, #19851 ) ;
#20935=ORIENTED_EDGE ( 'NONE', *, *, #17685, .T. ) ;
#20940=ORIENTED_EDGE ( 'NONE', *, *, #10203, .F. ) ;
#20949=CIRCLE ( 'NONE', #3720, 1.999999999999998224 ) ;
#20962=VECTOR ( 'NONE', #11952, 1000.000000000000000 ) ;
#20964=CIRCLE ( 'NONE', #3383, 4.199999999999997513 ) ;
#20984=DIRECTION ( 'NONE',  ( 0.01292394549866739996, 0.005513023399721131770, 0.9999012842304692006 ) ) ;
#20985=VECTOR ( 'NONE', #5978, 999.9999999999998863 ) ;
#20994=CARTESIAN_POINT ( 'NONE',  ( 43.22177362078638652, 125.3750519639578727, 249.0040540354910092 ) ) ;
#20996=DIRECTION ( 'NONE',  ( 7.125109674161246868E-05, -0.9999848031710253382, 0.005512562950850155054 ) ) ;
#21004=VERTEX_POINT ( 'NONE', #520 ) ;
#21007=CARTESIAN_POINT ( 'NONE',  ( 51.06003536384874053, 189.6011917897851333, -73.05933252543843537 ) ) ;
#21009=EDGE_CURVE ( 'NONE', #20773, #8421, #19232, .T. ) ;
#21010=CARTESIAN_POINT ( 'NONE',  ( 49.56102085612021568, 109.7790983012155834, -47.31406271648155837 ) ) ;
#21021=ORIENTED_EDGE ( 'NONE', *, *, #8252, .F. ) ;
#21024=CARTESIAN_POINT ( 'NONE',  ( -36.77797314829808784, 121.7015652700167152, 249.5406332993740648 ) ) ;
#21030=AXIS2_PLACEMENT_3D ( 'NONE', #22088, #17080, #18886 ) ;
#21039=ORIENTED_EDGE ( 'NONE', *, *, #4431, .F. ) ;
#21043=CYLINDRICAL_SURFACE ( 'NONE', #11533, 3.399999999999985700 ) ;
#21054=CARTESIAN_POINT ( 'NONE',  ( -36.79739265342710297, 125.3640259171584290, 248.0381828194013849 ) ) ;
#21058=ADVANCED_FACE ( 'NONE', ( #11082 ), #870, .F. ) ;
#21059=VECTOR ( 'NONE', #20180, 999.9999999999998863 ) ;
#21061=ORIENTED_EDGE ( 'NONE', *, *, #22183, .T. ) ;
#21065=CONICAL_SURFACE ( 'NONE', #18499, 3.399999999999985700, 1.029744258676653201 ) ;
#21068=CARTESIAN_POINT ( 'NONE',  ( -38.90465531275731337, 97.20110498407991884, 83.98952174397253145 ) ) ;
#21078=EDGE_LOOP ( 'NONE', ( #9025, #15843, #3574, #74 ) ) ;
#21088=DIRECTION ( 'NONE',  ( -0.01292394549866740169, -0.005513023399721063249, -0.9999012842304692006 ) ) ;
#21103=ORIENTED_EDGE ( 'NONE', *, *, #1441, .F. ) ;
#21105=EDGE_CURVE ( 'NONE', #22542, #848, #13646, .T. ) ;
#21120=CARTESIAN_POINT ( 'NONE',  ( -66.42677970909001317, 189.3893605493459233, -109.9672025422466959 ) ) ;
#21132=PLANE ( 'NONE',  #1961 ) ;
#21136=VERTEX_POINT ( 'NONE', #20017 ) ;
#21137=ADVANCED_FACE ( 'NONE', ( #11305 ), #8846, .F. ) ;
#21143=ORIENTED_EDGE ( 'NONE', *, *, #10071, .T. ) ;
#21145=DIRECTION ( 'NONE',  ( 0.01292394549866737220, 0.005513023399721000799, 0.9999012842304692006 ) ) ;
#21153=DIRECTION ( 'NONE',  ( 0.01292394549866740169, 0.005513023399720822990, 0.9999012842304693116 ) ) ;
#21154=CARTESIAN_POINT ( 'NONE',  ( -64.99457118636313169, 170.0000000000000284, 0.8400692238016805868 ) ) ;
#21157=CARTESIAN_POINT ( 'NONE',  ( -64.99143613810649356, 126.0006686604749291, 1.082621993639087288 ) ) ;
#21159=EDGE_LOOP ( 'NONE', ( #9923, #16054, #14676, #12950 ) ) ;
#21160=FACE_OUTER_BOUND ( 'NONE', #15589, .T. ) ;
#21161=FILL_AREA_STYLE ('',( #14183 ) ) ;
#21170=EDGE_CURVE ( 'NONE', #6519, #2719, #20949, .T. ) ;
#21176=CARTESIAN_POINT ( 'NONE',  ( -38.92003986412552052, 97.39926864640102622, 83.81297216957182172 ) ) ;
#21183=ADVANCED_FACE ( 'NONE', ( #11761 ), #11990, .F. ) ;
#21201=FACE_OUTER_BOUND ( 'NONE', #5828, .T. ) ;
#21203=EDGE_CURVE ( 'NONE', #6548, #13285, #8407, .T. ) ;
#21223=CARTESIAN_POINT ( 'NONE',  ( 50.99361748650641601, 111.8657007576893960, -48.09684511357723835 ) ) ;
#21228=CARTESIAN_POINT ( 'NONE',  ( -49.26352808811260786, 95.06875159149220167, -43.57455600632292914 ) ) ;
#21231=DIRECTION ( 'NONE',  ( 7.125109674141484573E-05, -0.9999848031710252272, 0.005512562950851785694 ) ) ;
#21237=VECTOR ( 'NONE', #9, 1000.000000000000114 ) ;
#21238=ORIENTED_EDGE ( 'NONE', *, *, #12170, .T. ) ;
#21248=LINE ( 'NONE', #17386, #5630 ) ;
#21249=ORIENTED_EDGE ( 'NONE', *, *, #21880, .T. ) ;
#21257=EDGE_CURVE ( 'NONE', #14285, #20578, #19522, .T. ) ;
#21262=CARTESIAN_POINT ( 'NONE',  ( -35.41327317553044907, 106.1692389898096280, 200.3757439048835920 ) ) ;
#21281=CARTESIAN_POINT ( 'NONE',  ( -38.90024297381467022, 95.59673886424684497, 82.77677384650711190 ) ) ;
#21287=AXIS2_PLACEMENT_3D ( 'NONE', #12935, #2577, #19904 ) ;
#21288=ADVANCED_FACE ( 'NONE', ( #606 ), #5749, .F. ) ;
#21298=ORIENTED_EDGE ( 'NONE', *, *, #8111, .F. ) ;
#21313=CARTESIAN_POINT ( 'NONE',  ( -40.94813932551373625, 95.97017003981163441, 82.42564028881616878 ) ) ;
#21316=DIRECTION ( 'NONE',  ( -0.01292394549866739996, -0.005513023399721131770, -0.9999012842304692006 ) ) ;
#21333=ADVANCED_FACE ( 'NONE', ( #11053, #13127 ), #5991, .F. ) ;
#21340=DIRECTION ( 'NONE',  ( 0.9999164797902017066, 6.965998958219365988E-18, -0.01292414190464157356 ) ) ;
#21346=DIRECTION ( 'NONE',  ( -0.01292394549866741384, -0.005513023399721118760, -0.9999012842304692006 ) ) ;
#21362=CARTESIAN_POINT ( 'NONE',  ( 40.98661049262742750, 104.0316351437719362, 76.07369909541560560 ) ) ;
#21365=DIRECTION ( 'NONE',  ( -0.9999164797902015955, -6.965998958219364448E-18, 0.01292414190464157182 ) ) ;
#21372=CARTESIAN_POINT ( 'NONE',  ( 49.10244780775150275, 189.5926834231606506, -74.57745705999737140 ) ) ;
#21378=CARTESIAN_POINT ( 'NONE',  ( -50.59410441606110709, 108.7350245882374224, -45.64162094458681196 ) ) ;
#21380=DIRECTION ( 'NONE',  ( -0.003413786507415475339, 0.9644842718275420390, -0.2641182225045781706 ) ) ;
#21388=EDGE_CURVE ( 'NONE', #8537, #21685, #21427, .T. ) ;
#21389=VERTEX_POINT ( 'NONE', #18417 ) ;
#21390=ORIENTED_EDGE ( 'NONE', *, *, #21388, .F. ) ;
#21399=DIRECTION ( 'NONE',  ( -0.9999164797902015955, -6.965998958219364448E-18, 0.01292414190464157182 ) ) ;
#21408=CARTESIAN_POINT ( 'NONE',  ( -45.67464185259402853, 168.2105890667581605, -51.90496219196452188 ) ) ;
#21415=VECTOR ( 'NONE', #18180, 1000.000000000000227 ) ;
#21416=EDGE_CURVE ( 'NONE', #19195, #7339, #5538, .T. ) ;
#21423=DIRECTION ( 'NONE',  ( -0.01292394549866695240, -0.005513023399718316314, -0.9999012842304693116 ) ) ;
#21424=CARTESIAN_POINT ( 'NONE',  ( 49.03340997568240311, 189.5897628274961164, -75.10636390159697839 ) ) ;
#21427=B_SPLINE_CURVE_WITH_KNOTS ( 'NONE', 3,
 ( #19990, #2548, #9554, #11389, #951, #5888, #622, #21828, #4163, #20354, #13142, #14886, #2565, #11406 ),
 .UNSPECIFIED., .F., .F.,
 ( 4, 2, 2, 2, 2, 2, 4 ),
 ( -9.867989413304089735E-06, 0.0008231430655169662313, 0.001239648592982118581, 0.001656154120447271040, 0.002489165175377561212, 0.002905670702842706298, 0.003322176230307851384 ),
 .UNSPECIFIED. ) ;
#21433=CARTESIAN_POINT ( 'NONE',  ( 52.64951385222703095, 106.8152934070036224, 70.24943021328142834 ) ) ;
#21439=AXIS2_PLACEMENT_3D ( 'NONE', #10269, #20820, #17284 ) ;
#21445=LINE ( 'NONE', #5706, #8060 ) ;
#21448=EDGE_LOOP ( 'NONE', ( #18416, #17756, #15980 ) ) ;
#21452=CARTESIAN_POINT ( 'NONE',  ( 49.42906846900682893, 109.0956092834914557, -47.06454438088354664 ) ) ;
#21454=CARTESIAN_POINT ( 'NONE',  ( -45.96244189366829858, 171.4878726268958360, -74.17150848012535391 ) ) ;
#21458=CARTESIAN_POINT ( 'NONE',  ( -49.99582398951010731, 170.0000000000000284, 0.6462070952320568828 ) ) ;
#21460=CARTESIAN_POINT ( 'NONE',  ( -40.54224781076989359, 96.08381321950558629, -41.69419662078171029 ) ) ;
#21461=CARTESIAN_POINT ( 'NONE',  ( -40.54264932485133954, 123.7663955596447352, -41.72526100787018777 ) ) ;
#21462=ORIENTED_EDGE ( 'NONE', *, *, #11950, .T. ) ;
#21464=DIRECTION ( 'NONE',  ( -0.9999164797902015955, -6.965998958219364448E-18, 0.01292414190464157182 ) ) ;
#21467=CARTESIAN_POINT ( 'NONE',  ( 41.91269397665269736, 107.0042359879021632, 70.57355413301411318 ) ) ;
#21476=DIRECTION ( 'NONE',  ( -0.01292394549866739822, -0.005513023399720312981, -0.9999012842304692006 ) ) ;
#21478=ORIENTED_EDGE ( 'NONE', *, *, #18668, .F. ) ;
#21488=FACE_OUTER_BOUND ( 'NONE', #12551, .T. ) ;
#21489=DIRECTION ( 'NONE',  ( 0.9999164797902015955, 6.965998958219364448E-18, -0.01292414190464157182 ) ) ;
#21491=CARTESIAN_POINT ( 'NONE',  ( 40.83918162370624572, 106.3640148094703193, 92.25234674474768326 ) ) ;
#21494=ORIENTED_EDGE ( 'NONE', *, *, #21972, .F. ) ;
#21499=CARTESIAN_POINT ( 'NONE',  ( 39.45107005634390873, 96.08378987033916019, -42.72816790301998680 ) ) ;
#21501=DIRECTION ( 'NONE',  ( -0.01292394549866740169, -0.005513023399719847208, -0.9999012842304693116 ) ) ;
#21502=CARTESIAN_POINT ( 'NONE',  ( -37.96378961924382622, 94.67635697584128707, 83.69533418420149928 ) ) ;
#21522=DIRECTION ( 'NONE',  ( -7.125109674159588039E-05, 0.9999848031710253382, -0.005512562950848870491 ) ) ;
#21528=AXIS2_PLACEMENT_3D ( 'NONE', #21154, #9079, #17858 ) ;
#21529=CARTESIAN_POINT ( 'NONE',  ( 52.26505271951528897, 106.8780608862217605, 70.19009726951736639 ) ) ;
#21530=CARTESIAN_POINT ( 'NONE',  ( -45.67439959886510081, 164.8106407359766763, -51.88621947793163258 ) ) ;
#21541=CARTESIAN_POINT ( 'NONE',  ( 51.02636103669043166, 169.5865232450209703, -75.66465169632658672 ) ) ;
#21550=CARTESIAN_POINT ( 'NONE',  ( 50.50946076891578684, 111.5620289191883643, -47.97866760800079788 ) ) ;
#21552=DIRECTION ( 'NONE',  ( 0.01292394549866737741, 0.005513023399721125699, 0.9999012842304693116 ) ) ;
#21576=CARTESIAN_POINT ( 'NONE',  ( -49.99724901144494282, 189.9996960634205436, 0.5359558362150538269 ) ) ;
#21583=CARTESIAN_POINT ( 'NONE',  ( 49.03514658276407800, 189.5905036194994864, -74.97200588752639305 ) ) ;
#21587=CARTESIAN_POINT ( 'NONE',  ( 19.42556530730579567, 136.7551719540686008, -44.57217540897067920 ) ) ;
#21588=ADVANCED_FACE ( 'NONE', ( #9186 ), #7478, .F. ) ;
#21592=VECTOR ( 'NONE', #8467, 1000.000000000000114 ) ;
#21593=CARTESIAN_POINT ( 'NONE',  ( -51.40218462123966248, 189.4003865961453812, -108.1612621023553658 ) ) ;
#21596=CARTESIAN_POINT ( 'NONE',  ( 51.99565694909048830, 170.0000000000000284, -0.6720553790413839046 ) ) ;
#21597=ORIENTED_EDGE ( 'NONE', *, *, #4872, .T. ) ;
#21609=CARTESIAN_POINT ( 'NONE',  ( -37.84108139470004772, 94.62834100696746020, 83.74230054658565336 ) ) ;
#21614=AXIS2_PLACEMENT_3D ( 'NONE', #10768, #19594, #311 ) ;
#21616=CIRCLE ( 'NONE', #13586, 112.5000000000000142 ) ;
#21619=ORIENTED_EDGE ( 'NONE', *, *, #2050, .T. ) ;
#21624=CARTESIAN_POINT ( 'NONE',  ( -28.13117687807453038, -5.346239964818102486, -9.967962068994514979 ) ) ;
#21631=AXIS2_PLACEMENT_3D ( 'NONE', #16175, #9362, #415 ) ;
#21642=CARTESIAN_POINT ( 'NONE',  ( 39.18815798788130422, 105.5072037373731888, 91.67997329703011644 ) ) ;
#21643=ORIENTED_EDGE ( 'NONE', *, *, #4704, .F. ) ;
#21645=VERTEX_POINT ( 'NONE', #12544 ) ;
#21649=AXIS2_PLACEMENT_3D ( 'NONE', #10541, #6853, #22456 ) ;
#21650=VERTEX_POINT ( 'NONE', #19638 ) ;
#21654=AXIS2_PLACEMENT_3D ( 'NONE', #12966, #13396, #18137 ) ;
#21657=EDGE_LOOP ( 'NONE', ( #5312, #7343, #10530, #20212 ) ) ;
#21664=ORIENTED_EDGE ( 'NONE', *, *, #8921, .T. ) ;
#21673=EDGE_CURVE ( 'NONE', #3218, #19636, #7350, .T. ) ;
#21676=EDGE_LOOP ( 'NONE', ( #4203, #21298, #18500, #7566 ) ) ;
#21680=VECTOR ( 'NONE', #20179, 1000.000000000000114 ) ;
#21681=PLANE ( 'NONE',  #12297 ) ;
#21684=EDGE_CURVE ( 'NONE', #16738, #15010, #9626, .T. ) ;
#21685=VERTEX_POINT ( 'NONE', #17727 ) ;
#21686=VERTEX_POINT ( 'NONE', #4128 ) ;
#21687=ADVANCED_FACE ( 'NONE', ( #2310 ), #22025, .T. ) ;
#21690=CARTESIAN_POINT ( 'NONE',  ( -51.62794139783391500, 111.4615474418020682, -46.62154578428164342 ) ) ;
#21693=CIRCLE ( 'NONE', #7416, 75.00000000000002842 ) ;
#21700=ORIENTED_EDGE ( 'NONE', *, *, #22220, .T. ) ;
#21709=( NAMED_UNIT ( * ) SI_UNIT ( $, .STERADIAN. ) SOLID_ANGLE_UNIT ( ) );
#21712=B_SPLINE_CURVE_WITH_KNOTS ( 'NONE', 3,
 ( #6828, #8653, #4982, #15480, #17180, #11909, #22433, #6503, #13956, #18891, #15696, #20492, #13746, #5212, #3155, #13847 ),
 .UNSPECIFIED., .F., .F.,
 ( 4, 2, 2, 2, 2, 2, 2, 4 ),
 ( 0.000000000000000000, 0.0003976901483970908080, 0.0007953802967941816160, 0.001193070445191272370, 0.001590760593588363232, 0.001988450741985454094, 0.002386140890382544739, 0.003181521187176709550 ),
 .UNSPECIFIED. ) ;
#21716=AXIS2_PLACEMENT_3D ( 'NONE', #13786, #15631, #19387 ) ;
#21717=ORIENTED_EDGE ( 'NONE', *, *, #14013, .F. ) ;
#21722=ORIENTED_EDGE ( 'NONE', *, *, #10272, .T. ) ;
#21725=CYLINDRICAL_SURFACE ( 'NONE', #6330, 4.199999999999997513 ) ;
#21734=AXIS2_PLACEMENT_3D ( 'NONE', #14335, #16180, #22657 ) ;
#21741=CARTESIAN_POINT ( 'NONE',  ( 47.42520555988353692, 108.9831309495507838, -44.78095393139386005 ) ) ;
#21747=AXIS2_PLACEMENT_3D ( 'NONE', #14889, #7856, #13049 ) ;
#21748=PLANE ( 'NONE',  #12997 ) ;
#21751=LINE ( 'NONE', #11561, #3997 ) ;
#21754=CARTESIAN_POINT ( 'NONE',  ( -39.32379867999515710, 107.5575245709147225, 72.11031038871728072 ) ) ;
#21760=CARTESIAN_POINT ( 'NONE',  ( 49.28843399868946307, 189.4915746906123957, -92.92109297631797915 ) ) ;
#21766=VECTOR ( 'NONE', #546, 999.9999999999998863 ) ;
#21769=CARTESIAN_POINT ( 'NONE',  ( 0.002351286192456229947, 137.0005014953561897, 0.1819145773780327657 ) ) ;
#21772=ORIENTED_EDGE ( 'NONE', *, *, #21935, .F. ) ;
#21784=CARTESIAN_POINT ( 'NONE',  ( -42.56628114047011735, 94.99786382055523859, -43.54068532293076288 ) ) ;
#21788=DIRECTION ( 'NONE',  ( 7.125109674141484573E-05, -0.9999848031710252272, 0.005512562950851785694 ) ) ;
#21802=AXIS2_PLACEMENT_3D ( 'NONE', #2171, #21464, #5724 ) ;
#21803=FACE_OUTER_BOUND ( 'NONE', #13814, .T. ) ;
#21805=EDGE_LOOP ( 'NONE', ( #8840, #19168, #13890, #18201 ) ) ;
#21814=CARTESIAN_POINT ( 'NONE',  ( -52.41270905777618339, 111.9218655255082524, -46.78102551800296283 ) ) ;
#21818=EDGE_CURVE ( 'NONE', #13676, #22322, #2656, .T. ) ;
#21821=ORIENTED_EDGE ( 'NONE', *, *, #19870, .F. ) ;
#21828=CARTESIAN_POINT ( 'NONE',  ( -38.08586061832574643, 105.9452655173670905, 92.44882592006047162 ) ) ;
#21829=CARTESIAN_POINT ( 'NONE',  ( -10.85567112094788200, 105.6999953372425409, 127.2994028633183063 ) ) ;
#21840=CARTESIAN_POINT ( 'NONE',  ( -65.93019277160487945, 189.6011917897851333, -71.54720792259536211 ) ) ;
#21842=APPLICATION_CONTEXT ( 'automotive_design' ) ;
#21846=ORIENTED_EDGE ( 'NONE', *, *, #17285, .T. ) ;
#21850=CARTESIAN_POINT ( 'NONE',  ( 47.86793869886106734, 110.7138355817038615, -44.79621871236214048 ) ) ;
#21851=CARTESIAN_POINT ( 'NONE',  ( 63.76679636398969819, 169.4762627770265340, -95.83069122569631304 ) ) ;
#21853=LINE ( 'NONE', #4293, #12508 ) ;
#21855=CARTESIAN_POINT ( 'NONE',  ( 29.05310264022292799, 95.51270090492249665, 81.29561921768979005 ) ) ;
#21867=CARTESIAN_POINT ( 'NONE',  ( 48.81886788476170125, 189.4982446786774517, -91.70508077603835773 ) ) ;
#21872=AXIS2_PLACEMENT_3D ( 'NONE', #13684, #17229, #6333 ) ;
#21876=DIRECTION ( 'NONE',  ( -0.01292394549866695240, -0.005513023399725255208, -0.9999012842304693116 ) ) ;
#21878=DIRECTION ( 'NONE',  ( 0.9999164797902015955, 6.965998958219364448E-18, -0.01292414190464157182 ) ) ;
#21880=EDGE_CURVE ( 'NONE', #7401, #7916, #15411, .T. ) ;
#21883=VERTEX_POINT ( 'NONE', #15633 ) ;
#21884=DIRECTION ( 'NONE',  ( -0.01292394549866740343, -0.005513023399721215904, -0.9999012842304693116 ) ) ;
#21892=ORIENTED_EDGE ( 'NONE', *, *, #18668, .T. ) ;
#21894=FACE_OUTER_BOUND ( 'NONE', #21805, .T. ) ;
#21898=AXIS2_PLACEMENT_3D ( 'NONE', #22470, #1715, #6870 ) ;
#21899=ORIENTED_EDGE ( 'NONE', *, *, #12866, .T. ) ;
#21908=CARTESIAN_POINT ( 'NONE',  ( -51.39706450756224854, 113.2585145316183883, -43.52722682608234805 ) ) ;
#21911=DIRECTION ( 'NONE',  ( -0.01292394549866737220, -0.005513023399721000799, -0.9999012842304692006 ) ) ;
#21919=CARTESIAN_POINT ( 'NONE',  ( 48.79389705813401434, 169.4872888238259634, -93.63702652866572862 ) ) ;
#21922=DIRECTION ( 'NONE',  ( 7.125109674161246868E-05, -0.9999848031710252272, 0.005512562950850154186 ) ) ;
#21924=DIRECTION ( 'NONE',  ( 0.01292394549866739996, 0.005513023399721131770, 0.9999012842304692006 ) ) ;
#21926=ORIENTED_EDGE ( 'NONE', *, *, #18923, .T. ) ;
#21932=B_SPLINE_CURVE_WITH_KNOTS ( 'NONE', 3,
 ( #2472, #18317, #9822, #16629, #13403, #2708, #985, #6258, #4291, #879, #4185, #19915, #20374, #5911 ),
 .UNSPECIFIED., .F., .F.,
 ( 4, 2, 2, 2, 2, 2, 4 ),
 ( 0.0002285844881980661123, 0.001015112171707181982, 0.001801639855216298014, 0.002194903696970858849, 0.002588167538725419468, 0.002981431380479980520, 0.003374695222234541138 ),
 .UNSPECIFIED. ) ;
#21933=LINE ( 'NONE', #8589, #1997 ) ;
#21935=EDGE_CURVE ( 'NONE', #2060, #3864, #10338, .T. ) ;
#21950=EDGE_CURVE ( 'NONE', #13554, #22043, #10718, .T. ) ;
#21951=FACE_OUTER_BOUND ( 'NONE', #14181, .T. ) ;
#21954=ORIENTED_EDGE ( 'NONE', *, *, #18333, .T. ) ;
#21957=ORIENTED_EDGE ( 'NONE', *, *, #12149, .T. ) ;
#21958=CARTESIAN_POINT ( 'NONE',  ( 48.60410837317779453, 111.9941758084687109, -44.81279311089502926 ) ) ;
#21961=ORIENTED_EDGE ( 'NONE', *, *, #4872, .F. ) ;
#21966=EDGE_CURVE ( 'NONE', #13016, #883, #13557, .T. ) ;
#21969=CARTESIAN_POINT ( 'NONE',  ( 26.59130080239608773, 189.4003865961453812, -109.1693451709174099 ) ) ;
#21971=ORIENTED_EDGE ( 'NONE', *, *, #9747, .F. ) ;
#21972=EDGE_CURVE ( 'NONE', #20464, #665, #22010, .T. ) ;
#21975=DIRECTION ( 'NONE',  ( 0.9999164797902015955, 6.965998958219364448E-18, -0.01292414190464157182 ) ) ;
#21983=CARTESIAN_POINT ( 'NONE',  ( 48.82059446874842479, 189.4989811950858609, -91.57149822991706856 ) ) ;
#21984=VERTEX_POINT ( 'NONE', #20770 ) ;
#21988=ORIENTED_EDGE ( 'NONE', *, *, #13013, .F. ) ;
#21994=CARTESIAN_POINT ( 'NONE',  ( -64.99457118636311748, 170.0000000000008242, 0.8400692238025471159 ) ) ;
#21997=ADVANCED_FACE ( 'NONE', ( #6443 ), #13455, .F. ) ;
#22010=CIRCLE ( 'NONE', #12139, 75.00000000000002842 ) ;
#22014=ADVANCED_FACE ( 'NONE', ( #3436 ), #10557, .F. ) ;
#22017=CARTESIAN_POINT ( 'NONE',  ( -10.80139054985347968, 105.7231500355213853, 131.4989882570862676 ) ) ;
#22022=AXIS2_PLACEMENT_3D ( 'NONE', #19240, #19463, #15941 ) ;
#22025=CYLINDRICAL_SURFACE ( 'NONE', #3737, 2.000000000000001332 ) ;
#22026=FACE_OUTER_BOUND ( 'NONE', #4838, .T. ) ;
#22028=CYLINDRICAL_SURFACE ( 'NONE', #7557, 7.499999999999991118 ) ;
#22041=DIRECTION ( 'NONE',  ( -0.9999164797902015955, -6.965998958219364448E-18, 0.01292414190464157182 ) ) ;
#22043=VERTEX_POINT ( 'NONE', #7218 ) ;
#22046=DIRECTION ( 'NONE',  ( -0.01292394549866741904, -0.005513023399721091004, -0.9999012842304693116 ) ) ;
#22056=DIRECTION ( 'NONE',  ( 0.9999164797902015955, 6.965998958219364448E-18, -0.01292414190464157182 ) ) ;
#22065=DIRECTION ( 'NONE',  ( -0.9999164797902015955, -6.965998958219364448E-18, 0.01292414190464157182 ) ) ;
#22087=ADVANCED_FACE ( 'NONE', ( #3774 ), #13893, .T. ) ;
#22088=CARTESIAN_POINT ( 'NONE',  ( -41.15169610061244754, 101.1708071963161615, 65.90309081746964637 ) ) ;
#22091=CARTESIAN_POINT ( 'NONE',  ( 41.48434878520766489, 95.06228642946297214, 83.37923770918371247 ) ) ;
#22092=DIRECTION ( 'NONE',  ( 7.125109674159588039E-05, -0.9999848031710253382, 0.005512562950848870491 ) ) ;
#22101=DIRECTION ( 'NONE',  ( 7.125109673814330634E-05, -0.9999848031710252272, 0.005512562950850199289 ) ) ;
#22114=CARTESIAN_POINT ( 'NONE',  ( -40.54264932485133954, 123.7663955596447352, -41.72526100787018777 ) ) ;
#22115=EDGE_LOOP ( 'NONE', ( #14249, #1062, #4223, #22399 ) ) ;
#22116=VECTOR ( 'NONE', #4723, 1000.000000000000114 ) ;
#22123=DIRECTION ( 'NONE',  ( -0.01292394549866741384, -0.005513023399721118760, -0.9999012842304692006 ) ) ;
#22133=SPHERICAL_SURFACE ( 'NONE', #11155, 2.000000000000000000 ) ;
#22134=EDGE_LOOP ( 'NONE', ( #13009, #16767, #2474, #6139 ) ) ;
#22144=CARTESIAN_POINT ( 'NONE',  ( -52.45778058759690765, 111.9218655230933734, -46.78044295554445142 ) ) ;
#22151=DIRECTION ( 'NONE',  ( -0.01292394549866737220, -0.005513023399721000799, -0.9999012842304692006 ) ) ;
#22170=CARTESIAN_POINT ( 'NONE',  ( 14.04474127379322468, 113.6585260871128611, 119.4329391803669722 ) ) ;
#22178=ORIENTED_EDGE ( 'NONE', *, *, #14846, .F. ) ;
#22183=EDGE_CURVE ( 'NONE', #2480, #2415, #19275, .T. ) ;
#22184=ORIENTED_EDGE ( 'NONE', *, *, #10833, .F. ) ;
#22185=ADVANCED_FACE ( 'NONE', ( #10975 ), #8105, .F. ) ;
#22188=CARTESIAN_POINT ( 'NONE',  ( 64.31784532510161512, 144.7109461922390778, -53.19707257213011076 ) ) ;
#22195=CARTESIAN_POINT ( 'NONE',  ( 44.31784132852413194, 168.2105890667581605, -53.06813496338226344 ) ) ;
#22205=EDGE_CURVE ( 'NONE', #10176, #21645, #2922, .T. ) ;
#22220=EDGE_CURVE ( 'NONE', #12189, #22554, #21853, .T. ) ;
#22224=CARTESIAN_POINT ( 'NONE',  ( 51.00051314569309824, 169.5754971982215125, -77.66445426478755110 ) ) ;
#22228=EDGE_CURVE ( 'NONE', #20787, #13165, #7000, .T. ) ;
#22231=CARTESIAN_POINT ( 'NONE',  ( 14.23860045627323601, 113.7412214381086670, 134.4314584438239706 ) ) ;
#22248=CARTESIAN_POINT ( 'NONE',  ( -50.94500546255758167, 109.1391869842444322, -43.51035759812305059 ) ) ;
#22256=EDGE_CURVE ( 'NONE', #7056, #17777, #6271, .T. ) ;
#22259=DIRECTION ( 'NONE',  ( 0.01292394549866739996, 0.005513023399721131770, 0.9999012842304692006 ) ) ;
#22268=CYLINDRICAL_SURFACE ( 'NONE', #8494, 7.921742784567028295 ) ;
#22269=ORIENTED_EDGE ( 'NONE', *, *, #17103, .T. ) ;
#22274=ADVANCED_FACE ( 'NONE', ( #3256 ), #19459, .F. ) ;
#22284=CARTESIAN_POINT ( 'NONE',  ( -51.43203027167875518, 189.4933473607019607, -91.29769442758977505 ) ) ;
#22285=ADVANCED_FACE ( 'NONE', ( #10068 ), #9830, .T. ) ;
#22296=VERTEX_POINT ( 'NONE', #9945 ) ;
#22304=CARTESIAN_POINT ( 'NONE',  ( -34.79726985247908999, 121.2962013336460956, 248.0347590154626971 ) ) ;
#22305=LINE ( 'NONE', #1106, #7425 ) ;
#22307=FACE_OUTER_BOUND ( 'NONE', #8216, .T. ) ;
#22310=CARTESIAN_POINT ( 'NONE',  ( 52.91240873130399081, 106.8060942374655156, 70.25530070199208410 ) ) ;
#22311=DIRECTION ( 'NONE',  ( -0.01292394549866740169, -0.005513023399721131770, -0.9999012842304693116 ) ) ;
#22313=B_SPLINE_CURVE_WITH_KNOTS ( 'NONE', 3,
 ( #17149, #4718, #5059, #15228, #18863, #1203, #18638, #17054, #3127, #18968, #22284, #11643, #1317, #6690, #8197, #1421 ),
 .UNSPECIFIED., .F., .F.,
 ( 4, 2, 2, 2, 2, 2, 2, 4 ),
 ( 6.938893903907228378E-18, 0.0003951465896843917307, 0.0007902931793687765225, 0.001185439769053161152, 0.001580586358737546106, 0.002370879538106300186, 0.002766026127790658252, 0.003161172717475016318 ),
 .UNSPECIFIED. ) ;
#22315=VERTEX_POINT ( 'NONE', #22310 ) ;
#22318=AXIS2_PLACEMENT_3D ( 'NONE', #1011, #18351, #21876 ) ;
#22322=VERTEX_POINT ( 'NONE', #6275 ) ;
#22323=CARTESIAN_POINT ( 'NONE',  ( -66.42308629463825298, 169.3906321239456361, -109.6814500331617381 ) ) ;
#22325=EDGE_CURVE ( 'NONE', #7542, #3218, #22516, .T. ) ;
#22326=DIRECTION ( 'NONE',  ( -0.01292394549866744159, -0.005513023399721009472, -0.9999012842304692006 ) ) ;
#22329=AXIS2_PLACEMENT_3D ( 'NONE', #11534, #18535, #11640 ) ;
#22338=ORIENTED_EDGE ( 'NONE', *, *, #14483, .F. ) ;
#22341=DIRECTION ( 'NONE',  ( -0.9999164797902017066, -6.965998958219365988E-18, 0.01292414190464157356 ) ) ;
#22343=AXIS2_PLACEMENT_3D ( 'NONE', #20339, #6776, #13468 ) ;
#22357=CARTESIAN_POINT ( 'NONE',  ( -48.80698602204240188, 140.5066718483590762, 92.62435808135882098 ) ) ;
#22377=FACE_OUTER_BOUND ( 'NONE', #20885, .T. ) ;
#22378=DIRECTION ( 'NONE',  ( -0.01292394549866747802, -0.005513023399721269681, -0.9999012842304692006 ) ) ;
#22389=ORIENTED_EDGE ( 'NONE', *, *, #2047, .T. ) ;
#22396=LINE ( 'NONE', #11411, #8561 ) ;
#22399=ORIENTED_EDGE ( 'NONE', *, *, #17694, .F. ) ;
#22404=LINE ( 'NONE', #22188, #7598 ) ;
#22417=FACE_OUTER_BOUND ( 'NONE', #22134, .T. ) ;
#22419=CIRCLE ( 'NONE', #19132, 110.5324305509042233 ) ;
#22420=VERTEX_POINT ( 'NONE', #15904 ) ;
#22425=CARTESIAN_POINT ( 'NONE',  ( 39.45066905836480942, 123.7663955596447352, -42.75919236024152070 ) ) ;
#22430=CARTESIAN_POINT ( 'NONE',  ( 49.99582398951009310, 170.0000000000008242, -0.6462070952312342076 ) ) ;
#22432=CARTESIAN_POINT ( 'NONE',  ( -51.99565694909051672, 170.0000000000000284, 0.6720553790413400508 ) ) ;
#22433=CARTESIAN_POINT ( 'NONE',  ( -51.20141213521757351, 189.5954075083848238, -72.78685549352853457 ) ) ;
#22434=PLANE ( 'NONE',  #14333 ) ;
#22439=CARTESIAN_POINT ( 'NONE',  ( -40.33104288128404846, 94.48610424851698042, 83.91830964824988826 ) ) ;
#22452=FACE_OUTER_BOUND ( 'NONE', #9135, .T. ) ;
#22456=DIRECTION ( 'NONE',  ( -0.01292394549866737914, -0.005513023399721009472, -0.9999012842304692006 ) ) ;
#22460=CYLINDRICAL_SURFACE ( 'NONE', #14689, 3.399999999999985700 ) ;
#22468=EDGE_LOOP ( 'NONE', ( #17405, #6424, #16528, #1688 ) ) ;
#22470=CARTESIAN_POINT ( 'NONE',  ( 44.31784132852413194, 168.2105890667581605, -53.06813496338226344 ) ) ;
#22471=DIRECTION ( 'NONE',  ( 0.01292394549866737220, 0.005513023399721000799, 0.9999012842304692006 ) ) ;
#22478=CARTESIAN_POINT ( 'NONE',  ( -48.58807999359533625, 108.9796592258344390, -43.53994181459253099 ) ) ;
#22484=CARTESIAN_POINT ( 'NONE',  ( 48.82059446874842479, 189.4989811950858609, -91.57149822991706856 ) ) ;
#22490=ORIENTED_EDGE ( 'NONE', *, *, #13061, .F. ) ;
#22497=EDGE_LOOP ( 'NONE', ( #7166, #14247, #6670, #11954 ) ) ;
#22501=ORIENTED_EDGE ( 'NONE', *, *, #12315, .F. ) ;
#22502=VECTOR ( 'NONE', #21346, 1000.000000000000114 ) ;
#22510=CARTESIAN_POINT ( 'NONE',  ( -40.33104288128404846, 94.48610424851698042, 83.91830964824988826 ) ) ;
#22516=B_SPLINE_CURVE_WITH_KNOTS ( 'NONE', 3,
 ( #16974, #8427, #6501, #13301, #16850, #17297, #1111, #10167, #8108, #22091, #6394, #8322, #18664, #17178 ),
 .UNSPECIFIED., .F., .F.,
 ( 4, 2, 2, 2, 2, 2, 4 ),
 ( 0.000000000000000000, 0.0003927847099521207183, 0.0007855694199042414366, 0.001178354129856362155, 0.001571138839808482873, 0.002356708259712697422, 0.003142277679616911536 ),
 .UNSPECIFIED. ) ;
#22526=ORIENTED_EDGE ( 'NONE', *, *, #4431, .T. ) ;
#22529=CARTESIAN_POINT ( 'NONE',  ( -49.10926328453583523, 107.8891387851018635, 70.20563931596009866 ) ) ;
#22538=DIRECTION ( 'NONE',  ( 0.009188991635466048358, -0.7031977391749438810, 0.7109349492407661675 ) ) ;
#22542=VERTEX_POINT ( 'NONE', #21919 ) ;
#22544=VERTEX_POINT ( 'NONE', #9425 ) ;
#22552=VERTEX_POINT ( 'NONE', #13465 ) ;
#22554=VERTEX_POINT ( 'NONE', #16585 ) ;
#22559=DIRECTION ( 'NONE',  ( -0.01292394549866740863, -0.005513023399721009472, -0.9999012842304692006 ) ) ;
#22564=LINE ( 'NONE', #3083, #10298 ) ;
#22574=CARTESIAN_POINT ( 'NONE',  ( 27.86414599017677673, -5.346239964818102486, -10.69171401565444235 ) ) ;
#22579=DIRECTION ( 'NONE',  ( -0.01292394549866743465, -0.005513023399721021615, -0.9999012842304692006 ) ) ;
#22584=CARTESIAN_POINT ( 'NONE',  ( -48.90524865575625313, 110.4369068636443671, -43.54387697287747727 ) ) ;
#22585=ORIENTED_EDGE ( 'NONE', *, *, #5205, .F. ) ;
#22592=DIRECTION ( 'NONE',  ( 0.01292394549866740169, 0.005513023399720822990, 0.9999012842304693116 ) ) ;
#22598=LINE ( 'NONE', #10575, #332 ) ;
#22602=ORIENTED_EDGE ( 'NONE', *, *, #14314, .T. ) ;
#22603=VERTEX_POINT ( 'NONE', #13124 ) ;
#22610=FACE_BOUND ( 'NONE', #10573, .T. ) ;
#22611=VERTEX_POINT ( 'NONE', #713 ) ;
#22617=FACE_OUTER_BOUND ( 'NONE', #11735, .T. ) ;
#22622=VERTEX_POINT ( 'NONE', #18286 ) ;
#22630=ADVANCED_FACE ( 'NONE', ( #835 ), #8041, .F. ) ;
#22633=CARTESIAN_POINT ( 'NONE',  ( -38.91888847133742502, 97.29933205984647770, 83.90205325766430633 ) ) ;
#22638=ORIENTED_EDGE ( 'NONE', *, *, #20293, .F. ) ;
#22648=ORIENTED_EDGE ( 'NONE', *, *, #12705, .T. ) ;
#22654=CARTESIAN_POINT ( 'NONE',  ( -26.94222022802838268, 95.51270090492249665, 82.01937116434972097 ) ) ;
#22656=ADVANCED_FACE ( 'NONE', ( #15310 ), #6662, .F. ) ;
#22657=DIRECTION ( 'NONE',  ( 0.01292394549866743465, 0.005513023399721021615, 0.9999012842304692006 ) ) ;
#22661=CARTESIAN_POINT ( 'NONE',  ( 14.08796030271276045, 105.6768406389637107, 122.7767139219343164 ) ) ;
ENDSEC;
END-ISO-10303-21;
